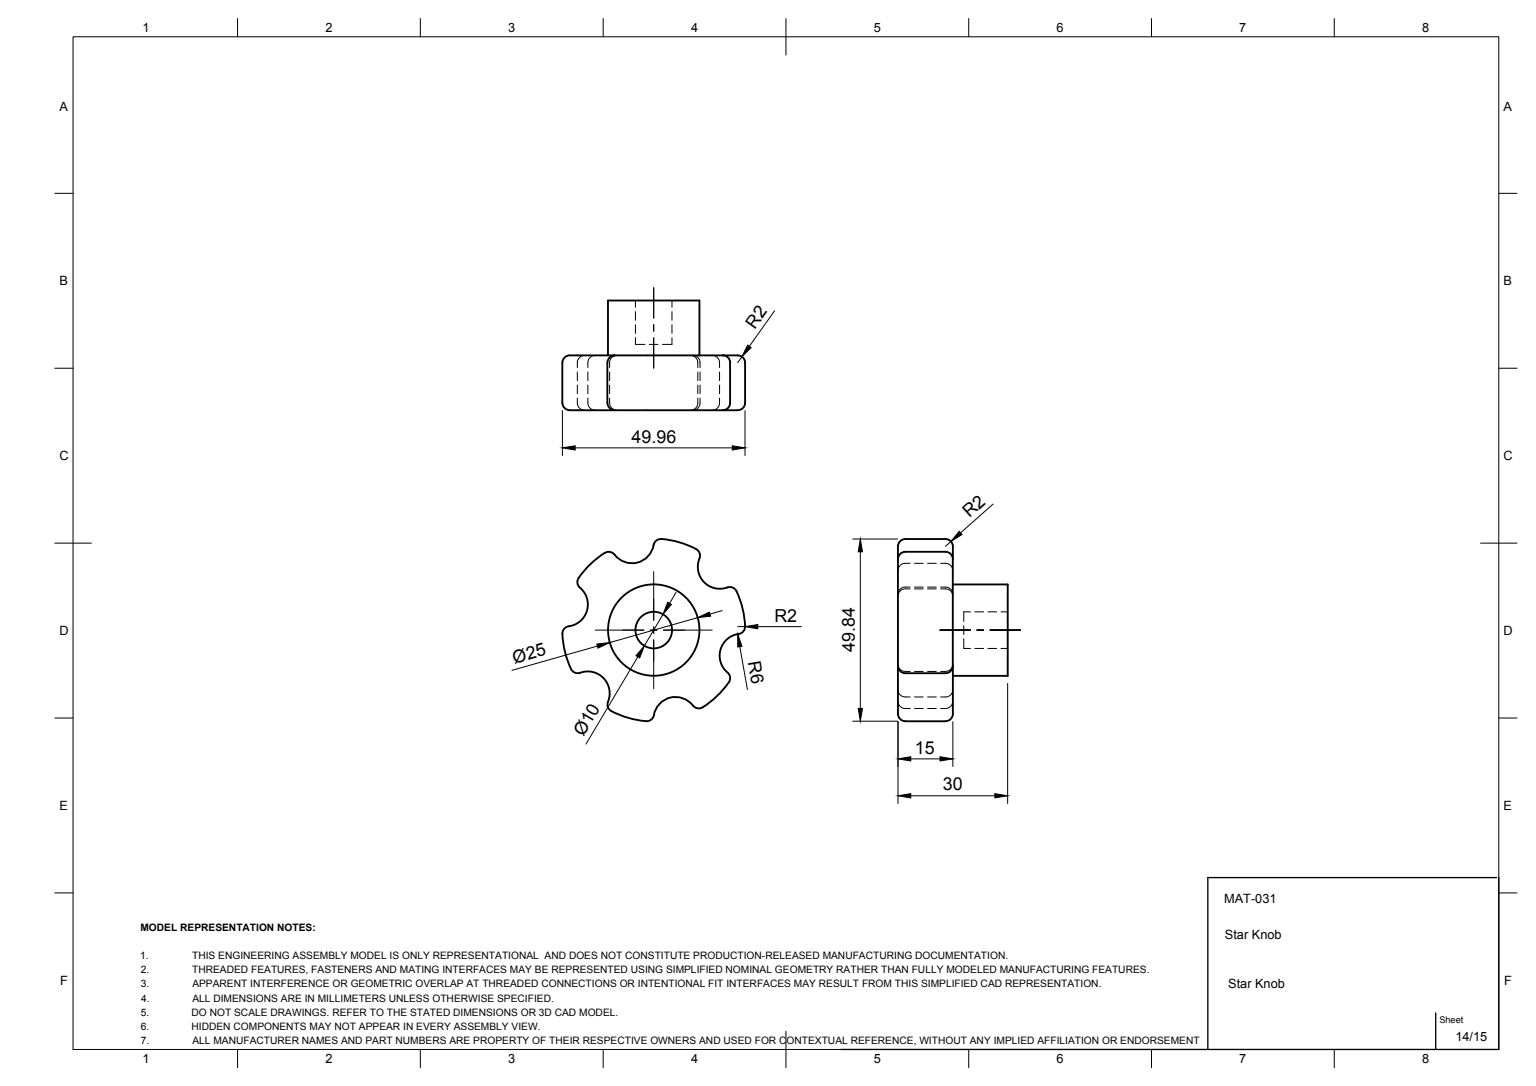
ISO-10303-21;
HEADER;
/* Generated by software containing ST-Developer
 * from STEP Tools, Inc. (www.steptools.com) 
 */

FILE_DESCRIPTION(
/* description */ ('STEP AP214'),
/* implementation_level */ '2;1');

FILE_NAME(
/* name */ 'Star Knob.step',
/* time_stamp */ '2026-11-14T06:58:01-08:00',
/* author */ (''),
/* organization */ (''),
/* preprocessor_version */ 'ST-DEVELOPER v20.2',
/* originating_system */ 'Autodesk Translation Framework v15.17.0.0',
/* authorisation */ '');

FILE_SCHEMA (('AUTOMOTIVE_DESIGN { 1 0 10303 214 3 1 1 }'));
ENDSEC;

DATA;
#10=MECHANICAL_DESIGN_GEOMETRIC_PRESENTATION_REPRESENTATION('',(#1158),#38635);
#93=SPHERICAL_SURFACE('',#18381,2.);
#94=SPHERICAL_SURFACE('',#18383,2.);
#95=SPHERICAL_SURFACE('',#18386,2.);
#96=SPHERICAL_SURFACE('',#18388,2.);
#97=SPHERICAL_SURFACE('',#18394,2.);
#98=SPHERICAL_SURFACE('',#18395,2.);
#99=SPHERICAL_SURFACE('',#18399,2.);
#100=SPHERICAL_SURFACE('',#18400,2.);
#101=SPHERICAL_SURFACE('',#18404,2.);
#102=SPHERICAL_SURFACE('',#18405,2.);
#103=SPHERICAL_SURFACE('',#18409,2.);
#104=SPHERICAL_SURFACE('',#18410,2.);
#105=SPHERICAL_SURFACE('',#18414,2.);
#106=SPHERICAL_SURFACE('',#18416,2.);
#107=SPHERICAL_SURFACE('',#18422,2.);
#108=SPHERICAL_SURFACE('',#18423,2.);
#109=SPHERICAL_SURFACE('',#18424,2.);
#110=SPHERICAL_SURFACE('',#18425,2.);
#111=SPHERICAL_SURFACE('',#18429,2.);
#112=SPHERICAL_SURFACE('',#18431,2.);
#113=SPHERICAL_SURFACE('',#18434,2.);
#114=SPHERICAL_SURFACE('',#18436,2.);
#115=SPHERICAL_SURFACE('',#18442,2.);
#116=SPHERICAL_SURFACE('',#18444,2.);
#155=TOROIDAL_SURFACE('',#18245,8.00000000000022,2.);
#156=TOROIDAL_SURFACE('',#18253,8.,2.);
#157=TOROIDAL_SURFACE('',#18258,8.00000000000095,2.);
#158=TOROIDAL_SURFACE('',#18266,8.00000000000152,2.);
#159=TOROIDAL_SURFACE('',#18274,8.00000000000143,2.);
#160=TOROIDAL_SURFACE('',#18279,8.00000000000082,2.);
#161=TOROIDAL_SURFACE('',#18314,23.,2.);
#162=TOROIDAL_SURFACE('',#18318,23.,2.);
#163=TOROIDAL_SURFACE('',#18322,23.,2.);
#164=TOROIDAL_SURFACE('',#18326,23.,2.);
#165=TOROIDAL_SURFACE('',#18330,23.,2.);
#166=TOROIDAL_SURFACE('',#18335,23.,2.);
#167=TOROIDAL_SURFACE('',#18339,23.,2.);
#168=TOROIDAL_SURFACE('',#18343,23.,2.);
#169=TOROIDAL_SURFACE('',#18347,23.,2.);
#170=TOROIDAL_SURFACE('',#18351,23.,2.);
#171=TOROIDAL_SURFACE('',#18369,23.,2.);
#172=TOROIDAL_SURFACE('',#18372,23.,2.);
#173=TOROIDAL_SURFACE('',#18384,8.00000000000082,2.);
#174=TOROIDAL_SURFACE('',#18397,8.00000000000143,2.);
#175=TOROIDAL_SURFACE('',#18407,8.00000000000152,2.);
#176=TOROIDAL_SURFACE('',#18411,8.00000000000095,2.);
#177=TOROIDAL_SURFACE('',#18433,8.,2.);
#178=TOROIDAL_SURFACE('',#18446,8.00000000000022,2.);
#883=FACE_BOUND('',#2951,.T.);
#884=FACE_BOUND('',#2953,.T.);
#1124=SHAPE_REPRESENTATION_RELATIONSHIP('SRR','None',#38697,#1138);
#1138=ADVANCED_BREP_SHAPE_REPRESENTATION('',(#1184),#38633);
#1158=STYLED_ITEM('',(#38765),#1184);
#1184=MANIFOLD_SOLID_BREP('Body1',#17624);
#1275=PLANE('',#18356);
#1276=PLANE('',#18362);
#1277=PLANE('',#18367);
#1278=PLANE('',#18368);
#1891=FACE_OUTER_BOUND('',#2918,.T.);
#1892=FACE_OUTER_BOUND('',#2919,.T.);
#1893=FACE_OUTER_BOUND('',#2920,.T.);
#1894=FACE_OUTER_BOUND('',#2921,.T.);
#1895=FACE_OUTER_BOUND('',#2922,.T.);
#1896=FACE_OUTER_BOUND('',#2923,.T.);
#1897=FACE_OUTER_BOUND('',#2924,.T.);
#1898=FACE_OUTER_BOUND('',#2925,.T.);
#1899=FACE_OUTER_BOUND('',#2926,.T.);
#1900=FACE_OUTER_BOUND('',#2927,.T.);
#1901=FACE_OUTER_BOUND('',#2928,.T.);
#1902=FACE_OUTER_BOUND('',#2929,.T.);
#1903=FACE_OUTER_BOUND('',#2930,.T.);
#1904=FACE_OUTER_BOUND('',#2931,.T.);
#1905=FACE_OUTER_BOUND('',#2932,.T.);
#1906=FACE_OUTER_BOUND('',#2933,.T.);
#1907=FACE_OUTER_BOUND('',#2934,.T.);
#1908=FACE_OUTER_BOUND('',#2935,.T.);
#1909=FACE_OUTER_BOUND('',#2936,.T.);
#1910=FACE_OUTER_BOUND('',#2937,.T.);
#1911=FACE_OUTER_BOUND('',#2938,.T.);
#1912=FACE_OUTER_BOUND('',#2939,.T.);
#1913=FACE_OUTER_BOUND('',#2940,.T.);
#1914=FACE_OUTER_BOUND('',#2941,.T.);
#1915=FACE_OUTER_BOUND('',#2942,.T.);
#1916=FACE_OUTER_BOUND('',#2943,.T.);
#1917=FACE_OUTER_BOUND('',#2944,.T.);
#1918=FACE_OUTER_BOUND('',#2945,.T.);
#1919=FACE_OUTER_BOUND('',#2946,.T.);
#1920=FACE_OUTER_BOUND('',#2947,.T.);
#1921=FACE_OUTER_BOUND('',#2948,.T.);
#1922=FACE_OUTER_BOUND('',#2949,.T.);
#1923=FACE_OUTER_BOUND('',#2950,.T.);
#1924=FACE_OUTER_BOUND('',#2952,.T.);
#1925=FACE_OUTER_BOUND('',#2954,.T.);
#1926=FACE_OUTER_BOUND('',#2955,.T.);
#1927=FACE_OUTER_BOUND('',#2956,.T.);
#1928=FACE_OUTER_BOUND('',#2957,.T.);
#1929=FACE_OUTER_BOUND('',#2958,.T.);
#1930=FACE_OUTER_BOUND('',#2959,.T.);
#1931=FACE_OUTER_BOUND('',#2960,.T.);
#1932=FACE_OUTER_BOUND('',#2961,.T.);
#1933=FACE_OUTER_BOUND('',#2962,.T.);
#1934=FACE_OUTER_BOUND('',#2963,.T.);
#1935=FACE_OUTER_BOUND('',#2964,.T.);
#1936=FACE_OUTER_BOUND('',#2965,.T.);
#1937=FACE_OUTER_BOUND('',#2966,.T.);
#1938=FACE_OUTER_BOUND('',#2967,.T.);
#1939=FACE_OUTER_BOUND('',#2968,.T.);
#1940=FACE_OUTER_BOUND('',#2969,.T.);
#1941=FACE_OUTER_BOUND('',#2970,.T.);
#1942=FACE_OUTER_BOUND('',#2971,.T.);
#1943=FACE_OUTER_BOUND('',#2972,.T.);
#1944=FACE_OUTER_BOUND('',#2973,.T.);
#1945=FACE_OUTER_BOUND('',#2974,.T.);
#1946=FACE_OUTER_BOUND('',#2975,.T.);
#1947=FACE_OUTER_BOUND('',#2976,.T.);
#1948=FACE_OUTER_BOUND('',#2977,.T.);
#1949=FACE_OUTER_BOUND('',#2978,.T.);
#1950=FACE_OUTER_BOUND('',#2979,.T.);
#1951=FACE_OUTER_BOUND('',#2980,.T.);
#1952=FACE_OUTER_BOUND('',#2981,.T.);
#1953=FACE_OUTER_BOUND('',#2982,.T.);
#1954=FACE_OUTER_BOUND('',#2983,.T.);
#1955=FACE_OUTER_BOUND('',#2984,.T.);
#1956=FACE_OUTER_BOUND('',#2985,.T.);
#1957=FACE_OUTER_BOUND('',#2986,.T.);
#1958=FACE_OUTER_BOUND('',#2987,.T.);
#1959=FACE_OUTER_BOUND('',#2988,.T.);
#1960=FACE_OUTER_BOUND('',#2989,.T.);
#1961=FACE_OUTER_BOUND('',#2990,.T.);
#1962=FACE_OUTER_BOUND('',#2991,.T.);
#1963=FACE_OUTER_BOUND('',#2992,.T.);
#1964=FACE_OUTER_BOUND('',#2993,.T.);
#1965=FACE_OUTER_BOUND('',#2994,.T.);
#1966=FACE_OUTER_BOUND('',#2995,.T.);
#1967=FACE_OUTER_BOUND('',#2996,.T.);
#1968=FACE_OUTER_BOUND('',#2997,.T.);
#2918=EDGE_LOOP('',(#12069,#12070,#12071,#12072));
#2919=EDGE_LOOP('',(#12073,#12074,#12075,#12076));
#2920=EDGE_LOOP('',(#12077,#12078,#12079,#12080));
#2921=EDGE_LOOP('',(#12081,#12082,#12083,#12084));
#2922=EDGE_LOOP('',(#12085,#12086,#12087,#12088));
#2923=EDGE_LOOP('',(#12089,#12090,#12091,#12092));
#2924=EDGE_LOOP('',(#12093,#12094,#12095,#12096));
#2925=EDGE_LOOP('',(#12097,#12098,#12099,#12100));
#2926=EDGE_LOOP('',(#12101,#12102,#12103,#12104));
#2927=EDGE_LOOP('',(#12105,#12106,#12107,#12108));
#2928=EDGE_LOOP('',(#12109,#12110,#12111,#12112));
#2929=EDGE_LOOP('',(#12113,#12114,#12115,#12116));
#2930=EDGE_LOOP('',(#12117,#12118,#12119,#12120));
#2931=EDGE_LOOP('',(#12121,#12122,#12123,#12124));
#2932=EDGE_LOOP('',(#12125,#12126,#12127,#12128));
#2933=EDGE_LOOP('',(#12129,#12130,#12131,#12132));
#2934=EDGE_LOOP('',(#12133,#12134,#12135,#12136));
#2935=EDGE_LOOP('',(#12137,#12138,#12139,#12140));
#2936=EDGE_LOOP('',(#12141,#12142,#12143,#12144));
#2937=EDGE_LOOP('',(#12145,#12146,#12147,#12148));
#2938=EDGE_LOOP('',(#12149,#12150,#12151,#12152));
#2939=EDGE_LOOP('',(#12153,#12154,#12155,#12156));
#2940=EDGE_LOOP('',(#12157,#12158,#12159,#12160));
#2941=EDGE_LOOP('',(#12161,#12162,#12163,#12164));
#2942=EDGE_LOOP('',(#12165,#12166,#12167,#12168));
#2943=EDGE_LOOP('',(#12169,#12170,#12171,#12172));
#2944=EDGE_LOOP('',(#12173,#12174,#12175,#12176));
#2945=EDGE_LOOP('',(#12177,#12178,#12179,#12180));
#2946=EDGE_LOOP('',(#12181,#12182,#12183,#12184));
#2947=EDGE_LOOP('',(#12185,#12186,#12187,#12188));
#2948=EDGE_LOOP('',(#12189,#12190,#12191,#12192,#12193,#12194,#12195,#12196,
#12197,#12198,#12199,#12200));
#2949=EDGE_LOOP('',(#12201,#12202,#12203,#12204));
#2950=EDGE_LOOP('',(#12205,#12206,#12207,#12208,#12209,#12210,#12211,#12212,
#12213,#12214,#12215,#12216));
#2951=EDGE_LOOP('',(#12217));
#2952=EDGE_LOOP('',(#12218));
#2953=EDGE_LOOP('',(#12219));
#2954=EDGE_LOOP('',(#12220));
#2955=EDGE_LOOP('',(#12221,#12222,#12223,#12224));
#2956=EDGE_LOOP('',(#12225,#12226,#12227,#12228));
#2957=EDGE_LOOP('',(#12229,#12230,#12231,#12232));
#2958=EDGE_LOOP('',(#12233,#12234,#12235,#12236));
#2959=EDGE_LOOP('',(#12237,#12238,#12239,#12240));
#2960=EDGE_LOOP('',(#12241,#12242,#12243));
#2961=EDGE_LOOP('',(#12244,#12245,#12246));
#2962=EDGE_LOOP('',(#12247,#12248,#12249,#12250));
#2963=EDGE_LOOP('',(#12251,#12252,#12253));
#2964=EDGE_LOOP('',(#12254,#12255,#12256));
#2965=EDGE_LOOP('',(#12257,#12258,#12259,#12260));
#2966=EDGE_LOOP('',(#12261,#12262,#12263,#12264));
#2967=EDGE_LOOP('',(#12265,#12266,#12267));
#2968=EDGE_LOOP('',(#12268,#12269,#12270));
#2969=EDGE_LOOP('',(#12271,#12272,#12273,#12274));
#2970=EDGE_LOOP('',(#12275,#12276,#12277));
#2971=EDGE_LOOP('',(#12278,#12279,#12280));
#2972=EDGE_LOOP('',(#12281,#12282,#12283,#12284));
#2973=EDGE_LOOP('',(#12285,#12286,#12287));
#2974=EDGE_LOOP('',(#12288,#12289,#12290));
#2975=EDGE_LOOP('',(#12291,#12292,#12293,#12294));
#2976=EDGE_LOOP('',(#12295,#12296,#12297));
#2977=EDGE_LOOP('',(#12298,#12299,#12300));
#2978=EDGE_LOOP('',(#12301,#12302,#12303,#12304));
#2979=EDGE_LOOP('',(#12305,#12306,#12307));
#2980=EDGE_LOOP('',(#12308,#12309,#12310));
#2981=EDGE_LOOP('',(#12311,#12312,#12313,#12314));
#2982=EDGE_LOOP('',(#12315,#12316,#12317,#12318));
#2983=EDGE_LOOP('',(#12319,#12320,#12321));
#2984=EDGE_LOOP('',(#12322,#12323,#12324));
#2985=EDGE_LOOP('',(#12325,#12326,#12327));
#2986=EDGE_LOOP('',(#12328,#12329,#12330));
#2987=EDGE_LOOP('',(#12331,#12332,#12333,#12334));
#2988=EDGE_LOOP('',(#12335,#12336,#12337));
#2989=EDGE_LOOP('',(#12338,#12339,#12340));
#2990=EDGE_LOOP('',(#12341,#12342,#12343,#12344));
#2991=EDGE_LOOP('',(#12345,#12346,#12347));
#2992=EDGE_LOOP('',(#12348,#12349,#12350));
#2993=EDGE_LOOP('',(#12351,#12352,#12353,#12354));
#2994=EDGE_LOOP('',(#12355,#12356,#12357,#12358));
#2995=EDGE_LOOP('',(#12359,#12360,#12361));
#2996=EDGE_LOOP('',(#12362,#12363,#12364));
#2997=EDGE_LOOP('',(#12365,#12366,#12367,#12368));
#3918=LINE('',#33069,#4862);
#3919=LINE('',#33072,#4863);
#3920=LINE('',#33095,#4864);
#3921=LINE('',#33098,#4865);
#3922=LINE('',#33112,#4866);
#3923=LINE('',#33115,#4867);
#3924=LINE('',#33138,#4868);
#3925=LINE('',#33140,#4869);
#3926=LINE('',#33143,#4870);
#3927=LINE('',#33147,#4871);
#3928=LINE('',#33151,#4872);
#3929=LINE('',#33154,#4873);
#3930=LINE('',#33159,#4874);
#3931=LINE('',#33165,#4875);
#3932=LINE('',#33172,#4876);
#3933=LINE('',#33175,#4877);
#3934=LINE('',#33180,#4878);
#3935=LINE('',#33189,#4879);
#3936=LINE('',#33196,#4880);
#3937=LINE('',#33199,#4881);
#3938=LINE('',#33262,#4882);
#3939=LINE('',#33263,#4883);
#3940=LINE('',#33281,#4884);
#3941=LINE('',#33284,#4885);
#3942=LINE('',#33287,#4886);
#3943=LINE('',#33291,#4887);
#4862=VECTOR('',#20893,1000.);
#4863=VECTOR('',#20896,1000.);
#4864=VECTOR('',#20921,1000.);
#4865=VECTOR('',#20924,1000.);
#4866=VECTOR('',#20939,1000.);
#4867=VECTOR('',#20942,1000.);
#4868=VECTOR('',#20967,1000.);
#4869=VECTOR('',#20970,1000.);
#4870=VECTOR('',#20973,1000.);
#4871=VECTOR('',#20978,1000.);
#4872=VECTOR('',#20983,1000.);
#4873=VECTOR('',#20986,1000.);
#4874=VECTOR('',#20991,5.);
#4875=VECTOR('',#20998,12.5);
#4876=VECTOR('',#21005,1000.);
#4877=VECTOR('',#21008,1000.);
#4878=VECTOR('',#21013,1000.);
#4879=VECTOR('',#21026,1000.);
#4880=VECTOR('',#21033,1000.);
#4881=VECTOR('',#21036,1000.);
#4882=VECTOR('',#21133,1000.);
#4883=VECTOR('',#21134,1000.);
#4884=VECTOR('',#21163,1000.);
#4885=VECTOR('',#21166,1000.);
#4886=VECTOR('',#21169,1000.);
#4887=VECTOR('',#21174,1000.);
#5795=CIRCLE('',#18246,6.00000000000022);
#5796=CIRCLE('',#18247,2.);
#5797=CIRCLE('',#18248,8.00000000000022);
#5798=CIRCLE('',#18249,2.);
#5799=CIRCLE('',#18251,2.);
#5800=CIRCLE('',#18252,2.);
#5801=CIRCLE('',#18254,6.);
#5802=CIRCLE('',#18255,2.);
#5803=CIRCLE('',#18256,8.);
#5804=CIRCLE('',#18257,2.);
#5805=CIRCLE('',#18259,6.00000000000095);
#5806=CIRCLE('',#18260,2.);
#5807=CIRCLE('',#18261,8.00000000000095);
#5808=CIRCLE('',#18262,2.);
#5809=CIRCLE('',#18264,2.);
#5810=CIRCLE('',#18265,2.);
#5811=CIRCLE('',#18267,6.00000000000152);
#5812=CIRCLE('',#18268,2.);
#5813=CIRCLE('',#18269,8.00000000000152);
#5814=CIRCLE('',#18270,2.);
#5815=CIRCLE('',#18272,2.);
#5816=CIRCLE('',#18273,2.);
#5817=CIRCLE('',#18275,6.00000000000143);
#5818=CIRCLE('',#18276,2.);
#5819=CIRCLE('',#18277,8.00000000000143);
#5820=CIRCLE('',#18278,2.);
#5821=CIRCLE('',#18280,6.00000000000081);
#5822=CIRCLE('',#18281,2.);
#5823=CIRCLE('',#18282,8.00000000000082);
#5824=CIRCLE('',#18283,2.);
#5825=CIRCLE('',#18285,2.);
#5826=CIRCLE('',#18286,2.);
#5827=CIRCLE('',#18288,6.00000000000143);
#5828=CIRCLE('',#18290,6.00000000000152);
#5829=CIRCLE('',#18292,6.00000000000095);
#5830=CIRCLE('',#18294,5.);
#5831=CIRCLE('',#18295,5.);
#5832=CIRCLE('',#18297,12.5);
#5833=CIRCLE('',#18298,12.5);
#5834=CIRCLE('',#18300,25.);
#5835=CIRCLE('',#18301,25.);
#5836=CIRCLE('',#18303,25.);
#5837=CIRCLE('',#18304,25.);
#5838=CIRCLE('',#18306,25.);
#5839=CIRCLE('',#18307,25.);
#5840=CIRCLE('',#18309,25.);
#5841=CIRCLE('',#18310,25.);
#5842=CIRCLE('',#18312,25.);
#5843=CIRCLE('',#18313,25.);
#5844=CIRCLE('',#18315,23.);
#5845=CIRCLE('',#18316,2.);
#5846=CIRCLE('',#18317,2.);
#5847=CIRCLE('',#18319,23.);
#5848=CIRCLE('',#18320,2.);
#5849=CIRCLE('',#18321,2.);
#5850=CIRCLE('',#18323,2.);
#5851=CIRCLE('',#18324,23.);
#5852=CIRCLE('',#18325,2.);
#5853=CIRCLE('',#18327,2.);
#5854=CIRCLE('',#18328,23.);
#5855=CIRCLE('',#18329,2.);
#5856=CIRCLE('',#18331,25.);
#5857=CIRCLE('',#18332,2.);
#5858=CIRCLE('',#18333,23.);
#5859=CIRCLE('',#18334,2.);
#5860=CIRCLE('',#18336,2.);
#5861=CIRCLE('',#18337,23.);
#5862=CIRCLE('',#18338,2.);
#5863=CIRCLE('',#18340,2.);
#5864=CIRCLE('',#18341,23.);
#5865=CIRCLE('',#18342,2.);
#5866=CIRCLE('',#18344,23.);
#5867=CIRCLE('',#18345,2.);
#5868=CIRCLE('',#18346,2.);
#5869=CIRCLE('',#18348,23.);
#5870=CIRCLE('',#18349,2.);
#5871=CIRCLE('',#18350,2.);
#5872=CIRCLE('',#18352,23.);
#5873=CIRCLE('',#18353,2.);
#5874=CIRCLE('',#18354,25.);
#5875=CIRCLE('',#18355,2.);
#5876=CIRCLE('',#18357,8.00000000000082);
#5877=CIRCLE('',#18358,8.);
#5878=CIRCLE('',#18359,8.00000000000022);
#5879=CIRCLE('',#18360,23.);
#5880=CIRCLE('',#18363,8.00000000000143);
#5881=CIRCLE('',#18364,8.00000000000151);
#5882=CIRCLE('',#18365,23.);
#5883=CIRCLE('',#18366,8.00000000000095);
#5884=CIRCLE('',#18370,2.);
#5885=CIRCLE('',#18371,2.);
#5886=CIRCLE('',#18373,2.);
#5887=CIRCLE('',#18374,2.);
#5888=CIRCLE('',#18376,6.00000000000022);
#5889=CIRCLE('',#18378,6.00000000000081);
#5890=CIRCLE('',#18380,6.);
#5891=CIRCLE('',#18382,2.);
#5892=CIRCLE('',#18385,2.);
#5893=CIRCLE('',#18387,2.);
#5894=CIRCLE('',#18389,2.);
#5895=CIRCLE('',#18392,2.);
#5896=CIRCLE('',#18393,2.);
#5897=CIRCLE('',#18396,2.);
#5898=CIRCLE('',#18398,2.);
#5899=CIRCLE('',#18402,2.);
#5900=CIRCLE('',#18403,2.);
#5901=CIRCLE('',#18406,2.);
#5902=CIRCLE('',#18408,2.);
#5903=CIRCLE('',#18412,2.);
#5904=CIRCLE('',#18413,2.);
#5905=CIRCLE('',#18415,2.);
#5906=CIRCLE('',#18417,2.);
#5907=CIRCLE('',#18419,2.);
#5908=CIRCLE('',#18421,2.);
#5909=CIRCLE('',#18426,2.);
#5910=CIRCLE('',#18428,2.);
#5911=CIRCLE('',#18430,2.);
#5912=CIRCLE('',#18432,2.);
#5913=CIRCLE('',#18435,2.);
#5914=CIRCLE('',#18437,2.);
#5915=CIRCLE('',#18439,2.);
#5916=CIRCLE('',#18441,2.);
#5917=CIRCLE('',#18443,2.);
#5918=CIRCLE('',#18445,2.);
#6885=VERTEX_POINT('',#33056);
#6886=VERTEX_POINT('',#33057);
#6887=VERTEX_POINT('',#33059);
#6888=VERTEX_POINT('',#33061);
#6889=VERTEX_POINT('',#33065);
#6890=VERTEX_POINT('',#33066);
#6891=VERTEX_POINT('',#33068);
#6892=VERTEX_POINT('',#33070);
#6893=VERTEX_POINT('',#33074);
#6894=VERTEX_POINT('',#33076);
#6895=VERTEX_POINT('',#33078);
#6896=VERTEX_POINT('',#33082);
#6897=VERTEX_POINT('',#33083);
#6898=VERTEX_POINT('',#33085);
#6899=VERTEX_POINT('',#33087);
#6900=VERTEX_POINT('',#33091);
#6901=VERTEX_POINT('',#33092);
#6902=VERTEX_POINT('',#33094);
#6903=VERTEX_POINT('',#33096);
#6904=VERTEX_POINT('',#33100);
#6905=VERTEX_POINT('',#33102);
#6906=VERTEX_POINT('',#33104);
#6907=VERTEX_POINT('',#33108);
#6908=VERTEX_POINT('',#33109);
#6909=VERTEX_POINT('',#33111);
#6910=VERTEX_POINT('',#33113);
#6911=VERTEX_POINT('',#33117);
#6912=VERTEX_POINT('',#33119);
#6913=VERTEX_POINT('',#33121);
#6914=VERTEX_POINT('',#33125);
#6915=VERTEX_POINT('',#33126);
#6916=VERTEX_POINT('',#33128);
#6917=VERTEX_POINT('',#33130);
#6918=VERTEX_POINT('',#33134);
#6919=VERTEX_POINT('',#33135);
#6920=VERTEX_POINT('',#33137);
#6921=VERTEX_POINT('',#33142);
#6922=VERTEX_POINT('',#33146);
#6923=VERTEX_POINT('',#33150);
#6924=VERTEX_POINT('',#33152);
#6925=VERTEX_POINT('',#33156);
#6926=VERTEX_POINT('',#33158);
#6927=VERTEX_POINT('',#33162);
#6928=VERTEX_POINT('',#33164);
#6929=VERTEX_POINT('',#33168);
#6930=VERTEX_POINT('',#33169);
#6931=VERTEX_POINT('',#33171);
#6932=VERTEX_POINT('',#33173);
#6933=VERTEX_POINT('',#33177);
#6934=VERTEX_POINT('',#33179);
#6935=VERTEX_POINT('',#33186);
#6936=VERTEX_POINT('',#33188);
#6937=VERTEX_POINT('',#33192);
#6938=VERTEX_POINT('',#33193);
#6939=VERTEX_POINT('',#33195);
#6940=VERTEX_POINT('',#33197);
#6941=VERTEX_POINT('',#33201);
#6942=VERTEX_POINT('',#33202);
#6943=VERTEX_POINT('',#33207);
#6944=VERTEX_POINT('',#33208);
#6945=VERTEX_POINT('',#33213);
#6946=VERTEX_POINT('',#33222);
#6947=VERTEX_POINT('',#33223);
#6948=VERTEX_POINT('',#33226);
#6949=VERTEX_POINT('',#33238);
#6950=VERTEX_POINT('',#33243);
#6951=VERTEX_POINT('',#33244);
#6952=VERTEX_POINT('',#33249);
#6953=VERTEX_POINT('',#33251);
#6954=VERTEX_POINT('',#33253);
#6955=VERTEX_POINT('',#33266);
#6956=VERTEX_POINT('',#33268);
#6957=VERTEX_POINT('',#33280);
#6958=VERTEX_POINT('',#33282);
#6959=VERTEX_POINT('',#33286);
#6960=VERTEX_POINT('',#33290);
#8821=EDGE_CURVE('',#6885,#6886,#5795,.T.);
#8822=EDGE_CURVE('',#6887,#6885,#5796,.T.);
#8823=EDGE_CURVE('',#6888,#6887,#5797,.T.);
#8824=EDGE_CURVE('',#6886,#6888,#5798,.T.);
#8825=EDGE_CURVE('',#6889,#6890,#5799,.T.);
#8826=EDGE_CURVE('',#6891,#6889,#3918,.T.);
#8827=EDGE_CURVE('',#6891,#6892,#5800,.T.);
#8828=EDGE_CURVE('',#6890,#6892,#3919,.T.);
#8829=EDGE_CURVE('',#6892,#6893,#5801,.T.);
#8830=EDGE_CURVE('',#6894,#6892,#5802,.T.);
#8831=EDGE_CURVE('',#6895,#6894,#5803,.T.);
#8832=EDGE_CURVE('',#6893,#6895,#5804,.T.);
#8833=EDGE_CURVE('',#6896,#6897,#5805,.T.);
#8834=EDGE_CURVE('',#6896,#6898,#5806,.T.);
#8835=EDGE_CURVE('',#6899,#6898,#5807,.T.);
#8836=EDGE_CURVE('',#6899,#6897,#5808,.T.);
#8837=EDGE_CURVE('',#6900,#6901,#5809,.T.);
#8838=EDGE_CURVE('',#6902,#6901,#3920,.T.);
#8839=EDGE_CURVE('',#6902,#6903,#5810,.T.);
#8840=EDGE_CURVE('',#6900,#6903,#3921,.T.);
#8841=EDGE_CURVE('',#6903,#6904,#5811,.T.);
#8842=EDGE_CURVE('',#6905,#6903,#5812,.T.);
#8843=EDGE_CURVE('',#6906,#6905,#5813,.T.);
#8844=EDGE_CURVE('',#6906,#6904,#5814,.T.);
#8845=EDGE_CURVE('',#6907,#6908,#5815,.T.);
#8846=EDGE_CURVE('',#6909,#6908,#3922,.T.);
#8847=EDGE_CURVE('',#6909,#6910,#5816,.T.);
#8848=EDGE_CURVE('',#6907,#6910,#3923,.T.);
#8849=EDGE_CURVE('',#6910,#6911,#5817,.T.);
#8850=EDGE_CURVE('',#6912,#6910,#5818,.T.);
#8851=EDGE_CURVE('',#6913,#6912,#5819,.T.);
#8852=EDGE_CURVE('',#6913,#6911,#5820,.T.);
#8853=EDGE_CURVE('',#6914,#6915,#5821,.T.);
#8854=EDGE_CURVE('',#6914,#6916,#5822,.T.);
#8855=EDGE_CURVE('',#6917,#6916,#5823,.T.);
#8856=EDGE_CURVE('',#6915,#6917,#5824,.T.);
#8857=EDGE_CURVE('',#6918,#6919,#5825,.T.);
#8858=EDGE_CURVE('',#6920,#6918,#3924,.T.);
#8859=EDGE_CURVE('',#6914,#6920,#5826,.T.);
#8860=EDGE_CURVE('',#6919,#6914,#3925,.T.);
#8861=EDGE_CURVE('',#6911,#6921,#3926,.T.);
#8862=EDGE_CURVE('',#6921,#6907,#5827,.T.);
#8863=EDGE_CURVE('',#6904,#6922,#3927,.T.);
#8864=EDGE_CURVE('',#6922,#6900,#5828,.T.);
#8865=EDGE_CURVE('',#6897,#6923,#3928,.T.);
#8866=EDGE_CURVE('',#6923,#6924,#5829,.T.);
#8867=EDGE_CURVE('',#6924,#6896,#3929,.T.);
#8868=EDGE_CURVE('',#6925,#6925,#5830,.T.);
#8869=EDGE_CURVE('',#6925,#6926,#3930,.T.);
#8870=EDGE_CURVE('',#6926,#6926,#5831,.T.);
#8871=EDGE_CURVE('',#6927,#6927,#5832,.T.);
#8872=EDGE_CURVE('',#6927,#6928,#3931,.T.);
#8873=EDGE_CURVE('',#6928,#6928,#5833,.T.);
#8874=EDGE_CURVE('',#6929,#6930,#5834,.T.);
#8875=EDGE_CURVE('',#6930,#6931,#3932,.T.);
#8876=EDGE_CURVE('',#6931,#6932,#5835,.T.);
#8877=EDGE_CURVE('',#6932,#6929,#3933,.T.);
#8878=EDGE_CURVE('',#6889,#6933,#5836,.T.);
#8879=EDGE_CURVE('',#6933,#6934,#3934,.T.);
#8880=EDGE_CURVE('',#6934,#6891,#5837,.T.);
#8881=EDGE_CURVE('',#6908,#6920,#5838,.T.);
#8882=EDGE_CURVE('',#6918,#6909,#5839,.T.);
#8883=EDGE_CURVE('',#6901,#6935,#5840,.T.);
#8884=EDGE_CURVE('',#6935,#6936,#3935,.T.);
#8885=EDGE_CURVE('',#6936,#6902,#5841,.T.);
#8886=EDGE_CURVE('',#6937,#6938,#5842,.T.);
#8887=EDGE_CURVE('',#6938,#6939,#3936,.T.);
#8888=EDGE_CURVE('',#6939,#6940,#5843,.T.);
#8889=EDGE_CURVE('',#6940,#6937,#3937,.T.);
#8890=EDGE_CURVE('',#6941,#6942,#5844,.T.);
#8891=EDGE_CURVE('',#6941,#6933,#5845,.T.);
#8892=EDGE_CURVE('',#6889,#6942,#5846,.T.);
#8893=EDGE_CURVE('',#6943,#6944,#5847,.T.);
#8894=EDGE_CURVE('',#6943,#6930,#5848,.T.);
#8895=EDGE_CURVE('',#6929,#6944,#5849,.T.);
#8896=EDGE_CURVE('',#6918,#6945,#5850,.T.);
#8897=EDGE_CURVE('',#6912,#6945,#5851,.T.);
#8898=EDGE_CURVE('',#6912,#6909,#5852,.T.);
#8899=EDGE_CURVE('',#6936,#6913,#5853,.T.);
#8900=EDGE_CURVE('',#6905,#6913,#5854,.T.);
#8901=EDGE_CURVE('',#6905,#6902,#5855,.T.);
#8902=EDGE_CURVE('',#6946,#6947,#5856,.T.);
#8903=EDGE_CURVE('',#6946,#6899,#5857,.T.);
#8904=EDGE_CURVE('',#6948,#6899,#5858,.T.);
#8905=EDGE_CURVE('',#6948,#6947,#5859,.T.);
#8906=EDGE_CURVE('',#6934,#6917,#5860,.T.);
#8907=EDGE_CURVE('',#6894,#6917,#5861,.T.);
#8908=EDGE_CURVE('',#6894,#6891,#5862,.T.);
#8909=EDGE_CURVE('',#6931,#6895,#5863,.T.);
#8910=EDGE_CURVE('',#6887,#6895,#5864,.T.);
#8911=EDGE_CURVE('',#6887,#6932,#5865,.T.);
#8912=EDGE_CURVE('',#6916,#6949,#5866,.T.);
#8913=EDGE_CURVE('',#6916,#6920,#5867,.T.);
#8914=EDGE_CURVE('',#6908,#6949,#5868,.T.);
#8915=EDGE_CURVE('',#6950,#6951,#5869,.T.);
#8916=EDGE_CURVE('',#6950,#6935,#5870,.T.);
#8917=EDGE_CURVE('',#6901,#6951,#5871,.T.);
#8918=EDGE_CURVE('',#6952,#6888,#5872,.T.);
#8919=EDGE_CURVE('',#6952,#6953,#5873,.T.);
#8920=EDGE_CURVE('',#6954,#6953,#5874,.T.);
#8921=EDGE_CURVE('',#6954,#6888,#5875,.T.);
#8922=EDGE_CURVE('',#6945,#6941,#5876,.T.);
#8923=EDGE_CURVE('',#6942,#6943,#5877,.T.);
#8924=EDGE_CURVE('',#6944,#6948,#5878,.T.);
#8925=EDGE_CURVE('',#6898,#6906,#5879,.T.);
#8926=EDGE_CURVE('',#6953,#6946,#3938,.T.);
#8927=EDGE_CURVE('',#6947,#6954,#3939,.T.);
#8928=EDGE_CURVE('',#6949,#6950,#5880,.T.);
#8929=EDGE_CURVE('',#6951,#6955,#5881,.T.);
#8930=EDGE_CURVE('',#6955,#6956,#5882,.T.);
#8931=EDGE_CURVE('',#6956,#6952,#5883,.T.);
#8932=EDGE_CURVE('',#6939,#6906,#5884,.T.);
#8933=EDGE_CURVE('',#6898,#6940,#5885,.T.);
#8934=EDGE_CURVE('',#6955,#6938,#5886,.T.);
#8935=EDGE_CURVE('',#6937,#6956,#5887,.T.);
#8936=EDGE_CURVE('',#6886,#6957,#3940,.T.);
#8937=EDGE_CURVE('',#6957,#6958,#5888,.T.);
#8938=EDGE_CURVE('',#6958,#6885,#3941,.T.);
#8939=EDGE_CURVE('',#6915,#6959,#3942,.T.);
#8940=EDGE_CURVE('',#6959,#6919,#5889,.T.);
#8941=EDGE_CURVE('',#6893,#6960,#3943,.T.);
#8942=EDGE_CURVE('',#6960,#6890,#5890,.T.);
#8943=EDGE_CURVE('',#6945,#6919,#5891,.T.);
#8944=EDGE_CURVE('',#6941,#6959,#5892,.T.);
#8945=EDGE_CURVE('',#6933,#6959,#5893,.T.);
#8946=EDGE_CURVE('',#6915,#6934,#5894,.T.);
#8947=EDGE_CURVE('',#6936,#6911,#5895,.T.);
#8948=EDGE_CURVE('',#6921,#6935,#5896,.T.);
#8949=EDGE_CURVE('',#6921,#6950,#5897,.T.);
#8950=EDGE_CURVE('',#6907,#6949,#5898,.T.);
#8951=EDGE_CURVE('',#6939,#6904,#5899,.T.);
#8952=EDGE_CURVE('',#6922,#6938,#5900,.T.);
#8953=EDGE_CURVE('',#6922,#6955,#5901,.T.);
#8954=EDGE_CURVE('',#6900,#6951,#5902,.T.);
#8955=EDGE_CURVE('',#6952,#6923,#5903,.T.);
#8956=EDGE_CURVE('',#6924,#6956,#5904,.T.);
#8957=EDGE_CURVE('',#6953,#6923,#5905,.T.);
#8958=EDGE_CURVE('',#6924,#6937,#5906,.T.);
#8959=EDGE_CURVE('',#6946,#6897,#5907,.T.);
#8960=EDGE_CURVE('',#6896,#6940,#5908,.T.);
#8961=EDGE_CURVE('',#6893,#6931,#5909,.T.);
#8962=EDGE_CURVE('',#6960,#6930,#5910,.T.);
#8963=EDGE_CURVE('',#6942,#6890,#5911,.T.);
#8964=EDGE_CURVE('',#6960,#6943,#5912,.T.);
#8965=EDGE_CURVE('',#6932,#6885,#5913,.T.);
#8966=EDGE_CURVE('',#6886,#6954,#5914,.T.);
#8967=EDGE_CURVE('',#6929,#6958,#5915,.T.);
#8968=EDGE_CURVE('',#6957,#6947,#5916,.T.);
#8969=EDGE_CURVE('',#6944,#6958,#5917,.T.);
#8970=EDGE_CURVE('',#6957,#6948,#5918,.T.);
#12069=ORIENTED_EDGE('',*,*,#8821,.F.);
#12070=ORIENTED_EDGE('',*,*,#8822,.F.);
#12071=ORIENTED_EDGE('',*,*,#8823,.F.);
#12072=ORIENTED_EDGE('',*,*,#8824,.F.);
#12073=ORIENTED_EDGE('',*,*,#8825,.F.);
#12074=ORIENTED_EDGE('',*,*,#8826,.F.);
#12075=ORIENTED_EDGE('',*,*,#8827,.T.);
#12076=ORIENTED_EDGE('',*,*,#8828,.F.);
#12077=ORIENTED_EDGE('',*,*,#8829,.F.);
#12078=ORIENTED_EDGE('',*,*,#8830,.F.);
#12079=ORIENTED_EDGE('',*,*,#8831,.F.);
#12080=ORIENTED_EDGE('',*,*,#8832,.F.);
#12081=ORIENTED_EDGE('',*,*,#8833,.F.);
#12082=ORIENTED_EDGE('',*,*,#8834,.T.);
#12083=ORIENTED_EDGE('',*,*,#8835,.F.);
#12084=ORIENTED_EDGE('',*,*,#8836,.T.);
#12085=ORIENTED_EDGE('',*,*,#8837,.T.);
#12086=ORIENTED_EDGE('',*,*,#8838,.F.);
#12087=ORIENTED_EDGE('',*,*,#8839,.T.);
#12088=ORIENTED_EDGE('',*,*,#8840,.F.);
#12089=ORIENTED_EDGE('',*,*,#8841,.F.);
#12090=ORIENTED_EDGE('',*,*,#8842,.F.);
#12091=ORIENTED_EDGE('',*,*,#8843,.F.);
#12092=ORIENTED_EDGE('',*,*,#8844,.T.);
#12093=ORIENTED_EDGE('',*,*,#8845,.T.);
#12094=ORIENTED_EDGE('',*,*,#8846,.F.);
#12095=ORIENTED_EDGE('',*,*,#8847,.T.);
#12096=ORIENTED_EDGE('',*,*,#8848,.F.);
#12097=ORIENTED_EDGE('',*,*,#8849,.F.);
#12098=ORIENTED_EDGE('',*,*,#8850,.F.);
#12099=ORIENTED_EDGE('',*,*,#8851,.F.);
#12100=ORIENTED_EDGE('',*,*,#8852,.T.);
#12101=ORIENTED_EDGE('',*,*,#8853,.F.);
#12102=ORIENTED_EDGE('',*,*,#8854,.T.);
#12103=ORIENTED_EDGE('',*,*,#8855,.F.);
#12104=ORIENTED_EDGE('',*,*,#8856,.F.);
#12105=ORIENTED_EDGE('',*,*,#8857,.F.);
#12106=ORIENTED_EDGE('',*,*,#8858,.F.);
#12107=ORIENTED_EDGE('',*,*,#8859,.F.);
#12108=ORIENTED_EDGE('',*,*,#8860,.F.);
#12109=ORIENTED_EDGE('',*,*,#8849,.T.);
#12110=ORIENTED_EDGE('',*,*,#8861,.T.);
#12111=ORIENTED_EDGE('',*,*,#8862,.T.);
#12112=ORIENTED_EDGE('',*,*,#8848,.T.);
#12113=ORIENTED_EDGE('',*,*,#8841,.T.);
#12114=ORIENTED_EDGE('',*,*,#8863,.T.);
#12115=ORIENTED_EDGE('',*,*,#8864,.T.);
#12116=ORIENTED_EDGE('',*,*,#8840,.T.);
#12117=ORIENTED_EDGE('',*,*,#8833,.T.);
#12118=ORIENTED_EDGE('',*,*,#8865,.T.);
#12119=ORIENTED_EDGE('',*,*,#8866,.T.);
#12120=ORIENTED_EDGE('',*,*,#8867,.T.);
#12121=ORIENTED_EDGE('',*,*,#8868,.F.);
#12122=ORIENTED_EDGE('',*,*,#8869,.T.);
#12123=ORIENTED_EDGE('',*,*,#8870,.T.);
#12124=ORIENTED_EDGE('',*,*,#8869,.F.);
#12125=ORIENTED_EDGE('',*,*,#8871,.F.);
#12126=ORIENTED_EDGE('',*,*,#8872,.T.);
#12127=ORIENTED_EDGE('',*,*,#8873,.T.);
#12128=ORIENTED_EDGE('',*,*,#8872,.F.);
#12129=ORIENTED_EDGE('',*,*,#8874,.T.);
#12130=ORIENTED_EDGE('',*,*,#8875,.T.);
#12131=ORIENTED_EDGE('',*,*,#8876,.T.);
#12132=ORIENTED_EDGE('',*,*,#8877,.T.);
#12133=ORIENTED_EDGE('',*,*,#8878,.T.);
#12134=ORIENTED_EDGE('',*,*,#8879,.T.);
#12135=ORIENTED_EDGE('',*,*,#8880,.T.);
#12136=ORIENTED_EDGE('',*,*,#8826,.T.);
#12137=ORIENTED_EDGE('',*,*,#8881,.T.);
#12138=ORIENTED_EDGE('',*,*,#8858,.T.);
#12139=ORIENTED_EDGE('',*,*,#8882,.T.);
#12140=ORIENTED_EDGE('',*,*,#8846,.T.);
#12141=ORIENTED_EDGE('',*,*,#8883,.T.);
#12142=ORIENTED_EDGE('',*,*,#8884,.T.);
#12143=ORIENTED_EDGE('',*,*,#8885,.T.);
#12144=ORIENTED_EDGE('',*,*,#8838,.T.);
#12145=ORIENTED_EDGE('',*,*,#8886,.T.);
#12146=ORIENTED_EDGE('',*,*,#8887,.T.);
#12147=ORIENTED_EDGE('',*,*,#8888,.T.);
#12148=ORIENTED_EDGE('',*,*,#8889,.T.);
#12149=ORIENTED_EDGE('',*,*,#8890,.F.);
#12150=ORIENTED_EDGE('',*,*,#8891,.T.);
#12151=ORIENTED_EDGE('',*,*,#8878,.F.);
#12152=ORIENTED_EDGE('',*,*,#8892,.T.);
#12153=ORIENTED_EDGE('',*,*,#8893,.F.);
#12154=ORIENTED_EDGE('',*,*,#8894,.T.);
#12155=ORIENTED_EDGE('',*,*,#8874,.F.);
#12156=ORIENTED_EDGE('',*,*,#8895,.T.);
#12157=ORIENTED_EDGE('',*,*,#8882,.F.);
#12158=ORIENTED_EDGE('',*,*,#8896,.T.);
#12159=ORIENTED_EDGE('',*,*,#8897,.F.);
#12160=ORIENTED_EDGE('',*,*,#8898,.T.);
#12161=ORIENTED_EDGE('',*,*,#8885,.F.);
#12162=ORIENTED_EDGE('',*,*,#8899,.T.);
#12163=ORIENTED_EDGE('',*,*,#8900,.F.);
#12164=ORIENTED_EDGE('',*,*,#8901,.T.);
#12165=ORIENTED_EDGE('',*,*,#8902,.F.);
#12166=ORIENTED_EDGE('',*,*,#8903,.T.);
#12167=ORIENTED_EDGE('',*,*,#8904,.F.);
#12168=ORIENTED_EDGE('',*,*,#8905,.T.);
#12169=ORIENTED_EDGE('',*,*,#8880,.F.);
#12170=ORIENTED_EDGE('',*,*,#8906,.T.);
#12171=ORIENTED_EDGE('',*,*,#8907,.F.);
#12172=ORIENTED_EDGE('',*,*,#8908,.T.);
#12173=ORIENTED_EDGE('',*,*,#8876,.F.);
#12174=ORIENTED_EDGE('',*,*,#8909,.T.);
#12175=ORIENTED_EDGE('',*,*,#8910,.F.);
#12176=ORIENTED_EDGE('',*,*,#8911,.T.);
#12177=ORIENTED_EDGE('',*,*,#8912,.F.);
#12178=ORIENTED_EDGE('',*,*,#8913,.T.);
#12179=ORIENTED_EDGE('',*,*,#8881,.F.);
#12180=ORIENTED_EDGE('',*,*,#8914,.T.);
#12181=ORIENTED_EDGE('',*,*,#8915,.F.);
#12182=ORIENTED_EDGE('',*,*,#8916,.T.);
#12183=ORIENTED_EDGE('',*,*,#8883,.F.);
#12184=ORIENTED_EDGE('',*,*,#8917,.T.);
#12185=ORIENTED_EDGE('',*,*,#8918,.F.);
#12186=ORIENTED_EDGE('',*,*,#8919,.T.);
#12187=ORIENTED_EDGE('',*,*,#8920,.F.);
#12188=ORIENTED_EDGE('',*,*,#8921,.T.);
#12189=ORIENTED_EDGE('',*,*,#8897,.T.);
#12190=ORIENTED_EDGE('',*,*,#8922,.T.);
#12191=ORIENTED_EDGE('',*,*,#8890,.T.);
#12192=ORIENTED_EDGE('',*,*,#8923,.T.);
#12193=ORIENTED_EDGE('',*,*,#8893,.T.);
#12194=ORIENTED_EDGE('',*,*,#8924,.T.);
#12195=ORIENTED_EDGE('',*,*,#8904,.T.);
#12196=ORIENTED_EDGE('',*,*,#8835,.T.);
#12197=ORIENTED_EDGE('',*,*,#8925,.T.);
#12198=ORIENTED_EDGE('',*,*,#8843,.T.);
#12199=ORIENTED_EDGE('',*,*,#8900,.T.);
#12200=ORIENTED_EDGE('',*,*,#8851,.T.);
#12201=ORIENTED_EDGE('',*,*,#8920,.T.);
#12202=ORIENTED_EDGE('',*,*,#8926,.T.);
#12203=ORIENTED_EDGE('',*,*,#8902,.T.);
#12204=ORIENTED_EDGE('',*,*,#8927,.T.);
#12205=ORIENTED_EDGE('',*,*,#8907,.T.);
#12206=ORIENTED_EDGE('',*,*,#8855,.T.);
#12207=ORIENTED_EDGE('',*,*,#8912,.T.);
#12208=ORIENTED_EDGE('',*,*,#8928,.T.);
#12209=ORIENTED_EDGE('',*,*,#8915,.T.);
#12210=ORIENTED_EDGE('',*,*,#8929,.T.);
#12211=ORIENTED_EDGE('',*,*,#8930,.T.);
#12212=ORIENTED_EDGE('',*,*,#8931,.T.);
#12213=ORIENTED_EDGE('',*,*,#8918,.T.);
#12214=ORIENTED_EDGE('',*,*,#8823,.T.);
#12215=ORIENTED_EDGE('',*,*,#8910,.T.);
#12216=ORIENTED_EDGE('',*,*,#8831,.T.);
#12217=ORIENTED_EDGE('',*,*,#8871,.T.);
#12218=ORIENTED_EDGE('',*,*,#8873,.F.);
#12219=ORIENTED_EDGE('',*,*,#8868,.T.);
#12220=ORIENTED_EDGE('',*,*,#8870,.F.);
#12221=ORIENTED_EDGE('',*,*,#8888,.F.);
#12222=ORIENTED_EDGE('',*,*,#8932,.T.);
#12223=ORIENTED_EDGE('',*,*,#8925,.F.);
#12224=ORIENTED_EDGE('',*,*,#8933,.T.);
#12225=ORIENTED_EDGE('',*,*,#8930,.F.);
#12226=ORIENTED_EDGE('',*,*,#8934,.T.);
#12227=ORIENTED_EDGE('',*,*,#8886,.F.);
#12228=ORIENTED_EDGE('',*,*,#8935,.T.);
#12229=ORIENTED_EDGE('',*,*,#8936,.T.);
#12230=ORIENTED_EDGE('',*,*,#8937,.T.);
#12231=ORIENTED_EDGE('',*,*,#8938,.T.);
#12232=ORIENTED_EDGE('',*,*,#8821,.T.);
#12233=ORIENTED_EDGE('',*,*,#8853,.T.);
#12234=ORIENTED_EDGE('',*,*,#8939,.T.);
#12235=ORIENTED_EDGE('',*,*,#8940,.T.);
#12236=ORIENTED_EDGE('',*,*,#8860,.T.);
#12237=ORIENTED_EDGE('',*,*,#8941,.T.);
#12238=ORIENTED_EDGE('',*,*,#8942,.T.);
#12239=ORIENTED_EDGE('',*,*,#8828,.T.);
#12240=ORIENTED_EDGE('',*,*,#8829,.T.);
#12241=ORIENTED_EDGE('',*,*,#8896,.F.);
#12242=ORIENTED_EDGE('',*,*,#8857,.T.);
#12243=ORIENTED_EDGE('',*,*,#8943,.F.);
#12244=ORIENTED_EDGE('',*,*,#8859,.T.);
#12245=ORIENTED_EDGE('',*,*,#8913,.F.);
#12246=ORIENTED_EDGE('',*,*,#8854,.F.);
#12247=ORIENTED_EDGE('',*,*,#8943,.T.);
#12248=ORIENTED_EDGE('',*,*,#8940,.F.);
#12249=ORIENTED_EDGE('',*,*,#8944,.F.);
#12250=ORIENTED_EDGE('',*,*,#8922,.F.);
#12251=ORIENTED_EDGE('',*,*,#8891,.F.);
#12252=ORIENTED_EDGE('',*,*,#8944,.T.);
#12253=ORIENTED_EDGE('',*,*,#8945,.F.);
#12254=ORIENTED_EDGE('',*,*,#8856,.T.);
#12255=ORIENTED_EDGE('',*,*,#8906,.F.);
#12256=ORIENTED_EDGE('',*,*,#8946,.F.);
#12257=ORIENTED_EDGE('',*,*,#8945,.T.);
#12258=ORIENTED_EDGE('',*,*,#8939,.F.);
#12259=ORIENTED_EDGE('',*,*,#8946,.T.);
#12260=ORIENTED_EDGE('',*,*,#8879,.F.);
#12261=ORIENTED_EDGE('',*,*,#8947,.F.);
#12262=ORIENTED_EDGE('',*,*,#8884,.F.);
#12263=ORIENTED_EDGE('',*,*,#8948,.F.);
#12264=ORIENTED_EDGE('',*,*,#8861,.F.);
#12265=ORIENTED_EDGE('',*,*,#8899,.F.);
#12266=ORIENTED_EDGE('',*,*,#8947,.T.);
#12267=ORIENTED_EDGE('',*,*,#8852,.F.);
#12268=ORIENTED_EDGE('',*,*,#8948,.T.);
#12269=ORIENTED_EDGE('',*,*,#8916,.F.);
#12270=ORIENTED_EDGE('',*,*,#8949,.F.);
#12271=ORIENTED_EDGE('',*,*,#8949,.T.);
#12272=ORIENTED_EDGE('',*,*,#8928,.F.);
#12273=ORIENTED_EDGE('',*,*,#8950,.F.);
#12274=ORIENTED_EDGE('',*,*,#8862,.F.);
#12275=ORIENTED_EDGE('',*,*,#8898,.F.);
#12276=ORIENTED_EDGE('',*,*,#8850,.T.);
#12277=ORIENTED_EDGE('',*,*,#8847,.F.);
#12278=ORIENTED_EDGE('',*,*,#8950,.T.);
#12279=ORIENTED_EDGE('',*,*,#8914,.F.);
#12280=ORIENTED_EDGE('',*,*,#8845,.F.);
#12281=ORIENTED_EDGE('',*,*,#8951,.F.);
#12282=ORIENTED_EDGE('',*,*,#8887,.F.);
#12283=ORIENTED_EDGE('',*,*,#8952,.F.);
#12284=ORIENTED_EDGE('',*,*,#8863,.F.);
#12285=ORIENTED_EDGE('',*,*,#8932,.F.);
#12286=ORIENTED_EDGE('',*,*,#8951,.T.);
#12287=ORIENTED_EDGE('',*,*,#8844,.F.);
#12288=ORIENTED_EDGE('',*,*,#8952,.T.);
#12289=ORIENTED_EDGE('',*,*,#8934,.F.);
#12290=ORIENTED_EDGE('',*,*,#8953,.F.);
#12291=ORIENTED_EDGE('',*,*,#8953,.T.);
#12292=ORIENTED_EDGE('',*,*,#8929,.F.);
#12293=ORIENTED_EDGE('',*,*,#8954,.F.);
#12294=ORIENTED_EDGE('',*,*,#8864,.F.);
#12295=ORIENTED_EDGE('',*,*,#8901,.F.);
#12296=ORIENTED_EDGE('',*,*,#8842,.T.);
#12297=ORIENTED_EDGE('',*,*,#8839,.F.);
#12298=ORIENTED_EDGE('',*,*,#8954,.T.);
#12299=ORIENTED_EDGE('',*,*,#8917,.F.);
#12300=ORIENTED_EDGE('',*,*,#8837,.F.);
#12301=ORIENTED_EDGE('',*,*,#8955,.F.);
#12302=ORIENTED_EDGE('',*,*,#8931,.F.);
#12303=ORIENTED_EDGE('',*,*,#8956,.F.);
#12304=ORIENTED_EDGE('',*,*,#8866,.F.);
#12305=ORIENTED_EDGE('',*,*,#8919,.F.);
#12306=ORIENTED_EDGE('',*,*,#8955,.T.);
#12307=ORIENTED_EDGE('',*,*,#8957,.F.);
#12308=ORIENTED_EDGE('',*,*,#8956,.T.);
#12309=ORIENTED_EDGE('',*,*,#8935,.F.);
#12310=ORIENTED_EDGE('',*,*,#8958,.F.);
#12311=ORIENTED_EDGE('',*,*,#8957,.T.);
#12312=ORIENTED_EDGE('',*,*,#8865,.F.);
#12313=ORIENTED_EDGE('',*,*,#8959,.F.);
#12314=ORIENTED_EDGE('',*,*,#8926,.F.);
#12315=ORIENTED_EDGE('',*,*,#8958,.T.);
#12316=ORIENTED_EDGE('',*,*,#8889,.F.);
#12317=ORIENTED_EDGE('',*,*,#8960,.F.);
#12318=ORIENTED_EDGE('',*,*,#8867,.F.);
#12319=ORIENTED_EDGE('',*,*,#8903,.F.);
#12320=ORIENTED_EDGE('',*,*,#8959,.T.);
#12321=ORIENTED_EDGE('',*,*,#8836,.F.);
#12322=ORIENTED_EDGE('',*,*,#8960,.T.);
#12323=ORIENTED_EDGE('',*,*,#8933,.F.);
#12324=ORIENTED_EDGE('',*,*,#8834,.F.);
#12325=ORIENTED_EDGE('',*,*,#8908,.F.);
#12326=ORIENTED_EDGE('',*,*,#8830,.T.);
#12327=ORIENTED_EDGE('',*,*,#8827,.F.);
#12328=ORIENTED_EDGE('',*,*,#8832,.T.);
#12329=ORIENTED_EDGE('',*,*,#8909,.F.);
#12330=ORIENTED_EDGE('',*,*,#8961,.F.);
#12331=ORIENTED_EDGE('',*,*,#8961,.T.);
#12332=ORIENTED_EDGE('',*,*,#8875,.F.);
#12333=ORIENTED_EDGE('',*,*,#8962,.F.);
#12334=ORIENTED_EDGE('',*,*,#8941,.F.);
#12335=ORIENTED_EDGE('',*,*,#8892,.F.);
#12336=ORIENTED_EDGE('',*,*,#8825,.T.);
#12337=ORIENTED_EDGE('',*,*,#8963,.F.);
#12338=ORIENTED_EDGE('',*,*,#8962,.T.);
#12339=ORIENTED_EDGE('',*,*,#8894,.F.);
#12340=ORIENTED_EDGE('',*,*,#8964,.F.);
#12341=ORIENTED_EDGE('',*,*,#8963,.T.);
#12342=ORIENTED_EDGE('',*,*,#8942,.F.);
#12343=ORIENTED_EDGE('',*,*,#8964,.T.);
#12344=ORIENTED_EDGE('',*,*,#8923,.F.);
#12345=ORIENTED_EDGE('',*,*,#8911,.F.);
#12346=ORIENTED_EDGE('',*,*,#8822,.T.);
#12347=ORIENTED_EDGE('',*,*,#8965,.F.);
#12348=ORIENTED_EDGE('',*,*,#8824,.T.);
#12349=ORIENTED_EDGE('',*,*,#8921,.F.);
#12350=ORIENTED_EDGE('',*,*,#8966,.F.);
#12351=ORIENTED_EDGE('',*,*,#8965,.T.);
#12352=ORIENTED_EDGE('',*,*,#8938,.F.);
#12353=ORIENTED_EDGE('',*,*,#8967,.F.);
#12354=ORIENTED_EDGE('',*,*,#8877,.F.);
#12355=ORIENTED_EDGE('',*,*,#8966,.T.);
#12356=ORIENTED_EDGE('',*,*,#8927,.F.);
#12357=ORIENTED_EDGE('',*,*,#8968,.F.);
#12358=ORIENTED_EDGE('',*,*,#8936,.F.);
#12359=ORIENTED_EDGE('',*,*,#8895,.F.);
#12360=ORIENTED_EDGE('',*,*,#8967,.T.);
#12361=ORIENTED_EDGE('',*,*,#8969,.F.);
#12362=ORIENTED_EDGE('',*,*,#8968,.T.);
#12363=ORIENTED_EDGE('',*,*,#8905,.F.);
#12364=ORIENTED_EDGE('',*,*,#8970,.F.);
#12365=ORIENTED_EDGE('',*,*,#8969,.T.);
#12366=ORIENTED_EDGE('',*,*,#8937,.F.);
#12367=ORIENTED_EDGE('',*,*,#8970,.T.);
#12368=ORIENTED_EDGE('',*,*,#8924,.F.);
#16349=CYLINDRICAL_SURFACE('',#18250,2.);
#16350=CYLINDRICAL_SURFACE('',#18263,2.);
#16351=CYLINDRICAL_SURFACE('',#18271,2.);
#16352=CYLINDRICAL_SURFACE('',#18284,2.);
#16353=CYLINDRICAL_SURFACE('',#18287,6.00000000000143);
#16354=CYLINDRICAL_SURFACE('',#18289,6.00000000000152);
#16355=CYLINDRICAL_SURFACE('',#18291,6.00000000000095);
#16356=CYLINDRICAL_SURFACE('',#18293,5.);
#16357=CYLINDRICAL_SURFACE('',#18296,12.5);
#16358=CYLINDRICAL_SURFACE('',#18299,25.);
#16359=CYLINDRICAL_SURFACE('',#18302,25.);
#16360=CYLINDRICAL_SURFACE('',#18305,25.);
#16361=CYLINDRICAL_SURFACE('',#18308,25.);
#16362=CYLINDRICAL_SURFACE('',#18311,25.);
#16363=CYLINDRICAL_SURFACE('',#18361,25.);
#16364=CYLINDRICAL_SURFACE('',#18375,6.00000000000022);
#16365=CYLINDRICAL_SURFACE('',#18377,6.00000000000081);
#16366=CYLINDRICAL_SURFACE('',#18379,6.);
#16367=CYLINDRICAL_SURFACE('',#18390,2.);
#16368=CYLINDRICAL_SURFACE('',#18391,2.);
#16369=CYLINDRICAL_SURFACE('',#18401,2.);
#16370=CYLINDRICAL_SURFACE('',#18418,2.);
#16371=CYLINDRICAL_SURFACE('',#18420,2.);
#16372=CYLINDRICAL_SURFACE('',#18427,2.);
#16373=CYLINDRICAL_SURFACE('',#18438,2.);
#16374=CYLINDRICAL_SURFACE('',#18440,2.);
#16850=ADVANCED_FACE('',(#1891),#155,.T.);
#16851=ADVANCED_FACE('',(#1892),#16349,.T.);
#16852=ADVANCED_FACE('',(#1893),#156,.T.);
#16853=ADVANCED_FACE('',(#1894),#157,.T.);
#16854=ADVANCED_FACE('',(#1895),#16350,.T.);
#16855=ADVANCED_FACE('',(#1896),#158,.T.);
#16856=ADVANCED_FACE('',(#1897),#16351,.T.);
#16857=ADVANCED_FACE('',(#1898),#159,.T.);
#16858=ADVANCED_FACE('',(#1899),#160,.T.);
#16859=ADVANCED_FACE('',(#1900),#16352,.T.);
#16860=ADVANCED_FACE('',(#1901),#16353,.F.);
#16861=ADVANCED_FACE('',(#1902),#16354,.F.);
#16862=ADVANCED_FACE('',(#1903),#16355,.F.);
#16863=ADVANCED_FACE('',(#1904),#16356,.F.);
#16864=ADVANCED_FACE('',(#1905),#16357,.T.);
#16865=ADVANCED_FACE('',(#1906),#16358,.T.);
#16866=ADVANCED_FACE('',(#1907),#16359,.T.);
#16867=ADVANCED_FACE('',(#1908),#16360,.T.);
#16868=ADVANCED_FACE('',(#1909),#16361,.T.);
#16869=ADVANCED_FACE('',(#1910),#16362,.T.);
#16870=ADVANCED_FACE('',(#1911),#161,.T.);
#16871=ADVANCED_FACE('',(#1912),#162,.T.);
#16872=ADVANCED_FACE('',(#1913),#163,.T.);
#16873=ADVANCED_FACE('',(#1914),#164,.T.);
#16874=ADVANCED_FACE('',(#1915),#165,.T.);
#16875=ADVANCED_FACE('',(#1916),#166,.T.);
#16876=ADVANCED_FACE('',(#1917),#167,.T.);
#16877=ADVANCED_FACE('',(#1918),#168,.T.);
#16878=ADVANCED_FACE('',(#1919),#169,.T.);
#16879=ADVANCED_FACE('',(#1920),#170,.T.);
#16880=ADVANCED_FACE('',(#1921),#1275,.F.);
#16881=ADVANCED_FACE('',(#1922),#16363,.T.);
#16882=ADVANCED_FACE('',(#1923,#883),#1276,.F.);
#16883=ADVANCED_FACE('',(#1924,#884),#1277,.F.);
#16884=ADVANCED_FACE('',(#1925),#1278,.F.);
#16885=ADVANCED_FACE('',(#1926),#171,.T.);
#16886=ADVANCED_FACE('',(#1927),#172,.T.);
#16887=ADVANCED_FACE('',(#1928),#16364,.F.);
#16888=ADVANCED_FACE('',(#1929),#16365,.F.);
#16889=ADVANCED_FACE('',(#1930),#16366,.F.);
#16890=ADVANCED_FACE('',(#1931),#93,.T.);
#16891=ADVANCED_FACE('',(#1932),#94,.T.);
#16892=ADVANCED_FACE('',(#1933),#173,.T.);
#16893=ADVANCED_FACE('',(#1934),#95,.T.);
#16894=ADVANCED_FACE('',(#1935),#96,.T.);
#16895=ADVANCED_FACE('',(#1936),#16367,.T.);
#16896=ADVANCED_FACE('',(#1937),#16368,.T.);
#16897=ADVANCED_FACE('',(#1938),#97,.T.);
#16898=ADVANCED_FACE('',(#1939),#98,.T.);
#16899=ADVANCED_FACE('',(#1940),#174,.T.);
#16900=ADVANCED_FACE('',(#1941),#99,.T.);
#16901=ADVANCED_FACE('',(#1942),#100,.T.);
#16902=ADVANCED_FACE('',(#1943),#16369,.T.);
#16903=ADVANCED_FACE('',(#1944),#101,.T.);
#16904=ADVANCED_FACE('',(#1945),#102,.T.);
#16905=ADVANCED_FACE('',(#1946),#175,.T.);
#16906=ADVANCED_FACE('',(#1947),#103,.T.);
#16907=ADVANCED_FACE('',(#1948),#104,.T.);
#16908=ADVANCED_FACE('',(#1949),#176,.T.);
#16909=ADVANCED_FACE('',(#1950),#105,.T.);
#16910=ADVANCED_FACE('',(#1951),#106,.T.);
#16911=ADVANCED_FACE('',(#1952),#16370,.T.);
#16912=ADVANCED_FACE('',(#1953),#16371,.T.);
#16913=ADVANCED_FACE('',(#1954),#107,.T.);
#16914=ADVANCED_FACE('',(#1955),#108,.T.);
#16915=ADVANCED_FACE('',(#1956),#109,.T.);
#16916=ADVANCED_FACE('',(#1957),#110,.T.);
#16917=ADVANCED_FACE('',(#1958),#16372,.T.);
#16918=ADVANCED_FACE('',(#1959),#111,.T.);
#16919=ADVANCED_FACE('',(#1960),#112,.T.);
#16920=ADVANCED_FACE('',(#1961),#177,.T.);
#16921=ADVANCED_FACE('',(#1962),#113,.T.);
#16922=ADVANCED_FACE('',(#1963),#114,.T.);
#16923=ADVANCED_FACE('',(#1964),#16373,.T.);
#16924=ADVANCED_FACE('',(#1965),#16374,.T.);
#16925=ADVANCED_FACE('',(#1966),#115,.T.);
#16926=ADVANCED_FACE('',(#1967),#116,.T.);
#16927=ADVANCED_FACE('',(#1968),#178,.T.);
#17624=CLOSED_SHELL('',(#16850,#16851,#16852,#16853,#16854,#16855,#16856,
#16857,#16858,#16859,#16860,#16861,#16862,#16863,#16864,#16865,#16866,#16867,
#16868,#16869,#16870,#16871,#16872,#16873,#16874,#16875,#16876,#16877,#16878,
#16879,#16880,#16881,#16882,#16883,#16884,#16885,#16886,#16887,#16888,#16889,
#16890,#16891,#16892,#16893,#16894,#16895,#16896,#16897,#16898,#16899,#16900,
#16901,#16902,#16903,#16904,#16905,#16906,#16907,#16908,#16909,#16910,#16911,
#16912,#16913,#16914,#16915,#16916,#16917,#16918,#16919,#16920,#16921,#16922,
#16923,#16924,#16925,#16926,#16927));
#18244=AXIS2_PLACEMENT_3D('',#33054,#20877,#20878);
#18245=AXIS2_PLACEMENT_3D('',#33055,#20879,#20880);
#18246=AXIS2_PLACEMENT_3D('',#33058,#20881,#20882);
#18247=AXIS2_PLACEMENT_3D('',#33060,#20883,#20884);
#18248=AXIS2_PLACEMENT_3D('',#33062,#20885,#20886);
#18249=AXIS2_PLACEMENT_3D('',#33063,#20887,#20888);
#18250=AXIS2_PLACEMENT_3D('',#33064,#20889,#20890);
#18251=AXIS2_PLACEMENT_3D('',#33067,#20891,#20892);
#18252=AXIS2_PLACEMENT_3D('',#33071,#20894,#20895);
#18253=AXIS2_PLACEMENT_3D('',#33073,#20897,#20898);
#18254=AXIS2_PLACEMENT_3D('',#33075,#20899,#20900);
#18255=AXIS2_PLACEMENT_3D('',#33077,#20901,#20902);
#18256=AXIS2_PLACEMENT_3D('',#33079,#20903,#20904);
#18257=AXIS2_PLACEMENT_3D('',#33080,#20905,#20906);
#18258=AXIS2_PLACEMENT_3D('',#33081,#20907,#20908);
#18259=AXIS2_PLACEMENT_3D('',#33084,#20909,#20910);
#18260=AXIS2_PLACEMENT_3D('',#33086,#20911,#20912);
#18261=AXIS2_PLACEMENT_3D('',#33088,#20913,#20914);
#18262=AXIS2_PLACEMENT_3D('',#33089,#20915,#20916);
#18263=AXIS2_PLACEMENT_3D('',#33090,#20917,#20918);
#18264=AXIS2_PLACEMENT_3D('',#33093,#20919,#20920);
#18265=AXIS2_PLACEMENT_3D('',#33097,#20922,#20923);
#18266=AXIS2_PLACEMENT_3D('',#33099,#20925,#20926);
#18267=AXIS2_PLACEMENT_3D('',#33101,#20927,#20928);
#18268=AXIS2_PLACEMENT_3D('',#33103,#20929,#20930);
#18269=AXIS2_PLACEMENT_3D('',#33105,#20931,#20932);
#18270=AXIS2_PLACEMENT_3D('',#33106,#20933,#20934);
#18271=AXIS2_PLACEMENT_3D('',#33107,#20935,#20936);
#18272=AXIS2_PLACEMENT_3D('',#33110,#20937,#20938);
#18273=AXIS2_PLACEMENT_3D('',#33114,#20940,#20941);
#18274=AXIS2_PLACEMENT_3D('',#33116,#20943,#20944);
#18275=AXIS2_PLACEMENT_3D('',#33118,#20945,#20946);
#18276=AXIS2_PLACEMENT_3D('',#33120,#20947,#20948);
#18277=AXIS2_PLACEMENT_3D('',#33122,#20949,#20950);
#18278=AXIS2_PLACEMENT_3D('',#33123,#20951,#20952);
#18279=AXIS2_PLACEMENT_3D('',#33124,#20953,#20954);
#18280=AXIS2_PLACEMENT_3D('',#33127,#20955,#20956);
#18281=AXIS2_PLACEMENT_3D('',#33129,#20957,#20958);
#18282=AXIS2_PLACEMENT_3D('',#33131,#20959,#20960);
#18283=AXIS2_PLACEMENT_3D('',#33132,#20961,#20962);
#18284=AXIS2_PLACEMENT_3D('',#33133,#20963,#20964);
#18285=AXIS2_PLACEMENT_3D('',#33136,#20965,#20966);
#18286=AXIS2_PLACEMENT_3D('',#33139,#20968,#20969);
#18287=AXIS2_PLACEMENT_3D('',#33141,#20971,#20972);
#18288=AXIS2_PLACEMENT_3D('',#33144,#20974,#20975);
#18289=AXIS2_PLACEMENT_3D('',#33145,#20976,#20977);
#18290=AXIS2_PLACEMENT_3D('',#33148,#20979,#20980);
#18291=AXIS2_PLACEMENT_3D('',#33149,#20981,#20982);
#18292=AXIS2_PLACEMENT_3D('',#33153,#20984,#20985);
#18293=AXIS2_PLACEMENT_3D('',#33155,#20987,#20988);
#18294=AXIS2_PLACEMENT_3D('',#33157,#20989,#20990);
#18295=AXIS2_PLACEMENT_3D('',#33160,#20992,#20993);
#18296=AXIS2_PLACEMENT_3D('',#33161,#20994,#20995);
#18297=AXIS2_PLACEMENT_3D('',#33163,#20996,#20997);
#18298=AXIS2_PLACEMENT_3D('',#33166,#20999,#21000);
#18299=AXIS2_PLACEMENT_3D('',#33167,#21001,#21002);
#18300=AXIS2_PLACEMENT_3D('',#33170,#21003,#21004);
#18301=AXIS2_PLACEMENT_3D('',#33174,#21006,#21007);
#18302=AXIS2_PLACEMENT_3D('',#33176,#21009,#21010);
#18303=AXIS2_PLACEMENT_3D('',#33178,#21011,#21012);
#18304=AXIS2_PLACEMENT_3D('',#33181,#21014,#21015);
#18305=AXIS2_PLACEMENT_3D('',#33182,#21016,#21017);
#18306=AXIS2_PLACEMENT_3D('',#33183,#21018,#21019);
#18307=AXIS2_PLACEMENT_3D('',#33184,#21020,#21021);
#18308=AXIS2_PLACEMENT_3D('',#33185,#21022,#21023);
#18309=AXIS2_PLACEMENT_3D('',#33187,#21024,#21025);
#18310=AXIS2_PLACEMENT_3D('',#33190,#21027,#21028);
#18311=AXIS2_PLACEMENT_3D('',#33191,#21029,#21030);
#18312=AXIS2_PLACEMENT_3D('',#33194,#21031,#21032);
#18313=AXIS2_PLACEMENT_3D('',#33198,#21034,#21035);
#18314=AXIS2_PLACEMENT_3D('',#33200,#21037,#21038);
#18315=AXIS2_PLACEMENT_3D('',#33203,#21039,#21040);
#18316=AXIS2_PLACEMENT_3D('',#33204,#21041,#21042);
#18317=AXIS2_PLACEMENT_3D('',#33205,#21043,#21044);
#18318=AXIS2_PLACEMENT_3D('',#33206,#21045,#21046);
#18319=AXIS2_PLACEMENT_3D('',#33209,#21047,#21048);
#18320=AXIS2_PLACEMENT_3D('',#33210,#21049,#21050);
#18321=AXIS2_PLACEMENT_3D('',#33211,#21051,#21052);
#18322=AXIS2_PLACEMENT_3D('',#33212,#21053,#21054);
#18323=AXIS2_PLACEMENT_3D('',#33214,#21055,#21056);
#18324=AXIS2_PLACEMENT_3D('',#33215,#21057,#21058);
#18325=AXIS2_PLACEMENT_3D('',#33216,#21059,#21060);
#18326=AXIS2_PLACEMENT_3D('',#33217,#21061,#21062);
#18327=AXIS2_PLACEMENT_3D('',#33218,#21063,#21064);
#18328=AXIS2_PLACEMENT_3D('',#33219,#21065,#21066);
#18329=AXIS2_PLACEMENT_3D('',#33220,#21067,#21068);
#18330=AXIS2_PLACEMENT_3D('',#33221,#21069,#21070);
#18331=AXIS2_PLACEMENT_3D('',#33224,#21071,#21072);
#18332=AXIS2_PLACEMENT_3D('',#33225,#21073,#21074);
#18333=AXIS2_PLACEMENT_3D('',#33227,#21075,#21076);
#18334=AXIS2_PLACEMENT_3D('',#33228,#21077,#21078);
#18335=AXIS2_PLACEMENT_3D('',#33229,#21079,#21080);
#18336=AXIS2_PLACEMENT_3D('',#33230,#21081,#21082);
#18337=AXIS2_PLACEMENT_3D('',#33231,#21083,#21084);
#18338=AXIS2_PLACEMENT_3D('',#33232,#21085,#21086);
#18339=AXIS2_PLACEMENT_3D('',#33233,#21087,#21088);
#18340=AXIS2_PLACEMENT_3D('',#33234,#21089,#21090);
#18341=AXIS2_PLACEMENT_3D('',#33235,#21091,#21092);
#18342=AXIS2_PLACEMENT_3D('',#33236,#21093,#21094);
#18343=AXIS2_PLACEMENT_3D('',#33237,#21095,#21096);
#18344=AXIS2_PLACEMENT_3D('',#33239,#21097,#21098);
#18345=AXIS2_PLACEMENT_3D('',#33240,#21099,#21100);
#18346=AXIS2_PLACEMENT_3D('',#33241,#21101,#21102);
#18347=AXIS2_PLACEMENT_3D('',#33242,#21103,#21104);
#18348=AXIS2_PLACEMENT_3D('',#33245,#21105,#21106);
#18349=AXIS2_PLACEMENT_3D('',#33246,#21107,#21108);
#18350=AXIS2_PLACEMENT_3D('',#33247,#21109,#21110);
#18351=AXIS2_PLACEMENT_3D('',#33248,#21111,#21112);
#18352=AXIS2_PLACEMENT_3D('',#33250,#21113,#21114);
#18353=AXIS2_PLACEMENT_3D('',#33252,#21115,#21116);
#18354=AXIS2_PLACEMENT_3D('',#33254,#21117,#21118);
#18355=AXIS2_PLACEMENT_3D('',#33255,#21119,#21120);
#18356=AXIS2_PLACEMENT_3D('',#33256,#21121,#21122);
#18357=AXIS2_PLACEMENT_3D('',#33257,#21123,#21124);
#18358=AXIS2_PLACEMENT_3D('',#33258,#21125,#21126);
#18359=AXIS2_PLACEMENT_3D('',#33259,#21127,#21128);
#18360=AXIS2_PLACEMENT_3D('',#33260,#21129,#21130);
#18361=AXIS2_PLACEMENT_3D('',#33261,#21131,#21132);
#18362=AXIS2_PLACEMENT_3D('',#33264,#21135,#21136);
#18363=AXIS2_PLACEMENT_3D('',#33265,#21137,#21138);
#18364=AXIS2_PLACEMENT_3D('',#33267,#21139,#21140);
#18365=AXIS2_PLACEMENT_3D('',#33269,#21141,#21142);
#18366=AXIS2_PLACEMENT_3D('',#33270,#21143,#21144);
#18367=AXIS2_PLACEMENT_3D('',#33271,#21145,#21146);
#18368=AXIS2_PLACEMENT_3D('',#33272,#21147,#21148);
#18369=AXIS2_PLACEMENT_3D('',#33273,#21149,#21150);
#18370=AXIS2_PLACEMENT_3D('',#33274,#21151,#21152);
#18371=AXIS2_PLACEMENT_3D('',#33275,#21153,#21154);
#18372=AXIS2_PLACEMENT_3D('',#33276,#21155,#21156);
#18373=AXIS2_PLACEMENT_3D('',#33277,#21157,#21158);
#18374=AXIS2_PLACEMENT_3D('',#33278,#21159,#21160);
#18375=AXIS2_PLACEMENT_3D('',#33279,#21161,#21162);
#18376=AXIS2_PLACEMENT_3D('',#33283,#21164,#21165);
#18377=AXIS2_PLACEMENT_3D('',#33285,#21167,#21168);
#18378=AXIS2_PLACEMENT_3D('',#33288,#21170,#21171);
#18379=AXIS2_PLACEMENT_3D('',#33289,#21172,#21173);
#18380=AXIS2_PLACEMENT_3D('',#33292,#21175,#21176);
#18381=AXIS2_PLACEMENT_3D('',#33293,#21177,#21178);
#18382=AXIS2_PLACEMENT_3D('',#33294,#21179,#21180);
#18383=AXIS2_PLACEMENT_3D('',#33295,#21181,#21182);
#18384=AXIS2_PLACEMENT_3D('',#33296,#21183,#21184);
#18385=AXIS2_PLACEMENT_3D('',#33297,#21185,#21186);
#18386=AXIS2_PLACEMENT_3D('',#33298,#21187,#21188);
#18387=AXIS2_PLACEMENT_3D('',#33299,#21189,#21190);
#18388=AXIS2_PLACEMENT_3D('',#33300,#21191,#21192);
#18389=AXIS2_PLACEMENT_3D('',#33301,#21193,#21194);
#18390=AXIS2_PLACEMENT_3D('',#33302,#21195,#21196);
#18391=AXIS2_PLACEMENT_3D('',#33303,#21197,#21198);
#18392=AXIS2_PLACEMENT_3D('',#33304,#21199,#21200);
#18393=AXIS2_PLACEMENT_3D('',#33305,#21201,#21202);
#18394=AXIS2_PLACEMENT_3D('',#33306,#21203,#21204);
#18395=AXIS2_PLACEMENT_3D('',#33307,#21205,#21206);
#18396=AXIS2_PLACEMENT_3D('',#33308,#21207,#21208);
#18397=AXIS2_PLACEMENT_3D('',#33309,#21209,#21210);
#18398=AXIS2_PLACEMENT_3D('',#33310,#21211,#21212);
#18399=AXIS2_PLACEMENT_3D('',#33311,#21213,#21214);
#18400=AXIS2_PLACEMENT_3D('',#33312,#21215,#21216);
#18401=AXIS2_PLACEMENT_3D('',#33313,#21217,#21218);
#18402=AXIS2_PLACEMENT_3D('',#33314,#21219,#21220);
#18403=AXIS2_PLACEMENT_3D('',#33315,#21221,#21222);
#18404=AXIS2_PLACEMENT_3D('',#33316,#21223,#21224);
#18405=AXIS2_PLACEMENT_3D('',#33317,#21225,#21226);
#18406=AXIS2_PLACEMENT_3D('',#33318,#21227,#21228);
#18407=AXIS2_PLACEMENT_3D('',#33319,#21229,#21230);
#18408=AXIS2_PLACEMENT_3D('',#33320,#21231,#21232);
#18409=AXIS2_PLACEMENT_3D('',#33321,#21233,#21234);
#18410=AXIS2_PLACEMENT_3D('',#33322,#21235,#21236);
#18411=AXIS2_PLACEMENT_3D('',#33323,#21237,#21238);
#18412=AXIS2_PLACEMENT_3D('',#33324,#21239,#21240);
#18413=AXIS2_PLACEMENT_3D('',#33325,#21241,#21242);
#18414=AXIS2_PLACEMENT_3D('',#33326,#21243,#21244);
#18415=AXIS2_PLACEMENT_3D('',#33327,#21245,#21246);
#18416=AXIS2_PLACEMENT_3D('',#33328,#21247,#21248);
#18417=AXIS2_PLACEMENT_3D('',#33329,#21249,#21250);
#18418=AXIS2_PLACEMENT_3D('',#33330,#21251,#21252);
#18419=AXIS2_PLACEMENT_3D('',#33331,#21253,#21254);
#18420=AXIS2_PLACEMENT_3D('',#33332,#21255,#21256);
#18421=AXIS2_PLACEMENT_3D('',#33333,#21257,#21258);
#18422=AXIS2_PLACEMENT_3D('',#33334,#21259,#21260);
#18423=AXIS2_PLACEMENT_3D('',#33335,#21261,#21262);
#18424=AXIS2_PLACEMENT_3D('',#33336,#21263,#21264);
#18425=AXIS2_PLACEMENT_3D('',#33337,#21265,#21266);
#18426=AXIS2_PLACEMENT_3D('',#33338,#21267,#21268);
#18427=AXIS2_PLACEMENT_3D('',#33339,#21269,#21270);
#18428=AXIS2_PLACEMENT_3D('',#33340,#21271,#21272);
#18429=AXIS2_PLACEMENT_3D('',#33341,#21273,#21274);
#18430=AXIS2_PLACEMENT_3D('',#33342,#21275,#21276);
#18431=AXIS2_PLACEMENT_3D('',#33343,#21277,#21278);
#18432=AXIS2_PLACEMENT_3D('',#33344,#21279,#21280);
#18433=AXIS2_PLACEMENT_3D('',#33345,#21281,#21282);
#18434=AXIS2_PLACEMENT_3D('',#33346,#21283,#21284);
#18435=AXIS2_PLACEMENT_3D('',#33347,#21285,#21286);
#18436=AXIS2_PLACEMENT_3D('',#33348,#21287,#21288);
#18437=AXIS2_PLACEMENT_3D('',#33349,#21289,#21290);
#18438=AXIS2_PLACEMENT_3D('',#33350,#21291,#21292);
#18439=AXIS2_PLACEMENT_3D('',#33351,#21293,#21294);
#18440=AXIS2_PLACEMENT_3D('',#33352,#21295,#21296);
#18441=AXIS2_PLACEMENT_3D('',#33353,#21297,#21298);
#18442=AXIS2_PLACEMENT_3D('',#33354,#21299,#21300);
#18443=AXIS2_PLACEMENT_3D('',#33355,#21301,#21302);
#18444=AXIS2_PLACEMENT_3D('',#33356,#21303,#21304);
#18445=AXIS2_PLACEMENT_3D('',#33357,#21305,#21306);
#18446=AXIS2_PLACEMENT_3D('',#33358,#21307,#21308);
#20877=DIRECTION('axis',(0.,0.,1.));
#20878=DIRECTION('refdir',(1.,0.,0.));
#20879=DIRECTION('center_axis',(-1.,-1.22464679914735E-16,0.));
#20880=DIRECTION('ref_axis',(1.77635683940021E-16,-1.,0.));
#20881=DIRECTION('center_axis',(1.,1.22464679914735E-16,0.));
#20882=DIRECTION('ref_axis',(1.22464679914735E-16,-1.,0.));
#20883=DIRECTION('center_axis',(0.,0.80466773100941,-0.593725393319309));
#20884=DIRECTION('ref_axis',(0.,0.593725393319309,0.80466773100941));
#20885=DIRECTION('center_axis',(-1.,-1.22464679914735E-16,0.));
#20886=DIRECTION('ref_axis',(1.22464679914735E-16,-1.,0.));
#20887=DIRECTION('center_axis',(-1.72383876846542E-15,0.111847407981753,
-0.993725393319383));
#20888=DIRECTION('ref_axis',(1.05814669609279E-32,0.993725393319383,0.111847407981753));
#20889=DIRECTION('center_axis',(1.,1.22464679914735E-16,0.));
#20890=DIRECTION('ref_axis',(-1.22464679914735E-16,1.,0.));
#20891=DIRECTION('center_axis',(-1.,-1.99493199737333E-16,-8.70659703262162E-17));
#20892=DIRECTION('ref_axis',(1.99493199737333E-16,-1.,-1.51035382683587E-33));
#20893=DIRECTION('',(-1.,-1.22464679914735E-16,0.));
#20894=DIRECTION('center_axis',(-1.,0.,0.));
#20895=DIRECTION('ref_axis',(0.,0.,1.));
#20896=DIRECTION('',(1.,1.22464679914735E-16,0.));
#20897=DIRECTION('center_axis',(-1.,-1.22464679914735E-16,0.));
#20898=DIRECTION('ref_axis',(1.77635683940025E-16,-1.,0.));
#20899=DIRECTION('center_axis',(1.,1.22464679914735E-16,0.));
#20900=DIRECTION('ref_axis',(1.22464679914735E-16,-1.,0.));
#20901=DIRECTION('center_axis',(0.,0.916515138991168,0.400000000000001));
#20902=DIRECTION('ref_axis',(0.,-0.400000000000001,0.916515138991168));
#20903=DIRECTION('center_axis',(-1.,-1.22464679914735E-16,0.));
#20904=DIRECTION('ref_axis',(1.22464679914735E-16,-1.,0.));
#20905=DIRECTION('center_axis',(-1.7347234759768E-16,0.916515138991168,
-0.399999999999999));
#20906=DIRECTION('ref_axis',(-1.38807035205952E-32,0.399999999999999,0.916515138991168));
#20907=DIRECTION('center_axis',(1.,1.22464679914735E-16,0.));
#20908=DIRECTION('ref_axis',(-1.33226762955006E-16,1.,0.));
#20909=DIRECTION('center_axis',(-1.,-1.22464679914735E-16,0.));
#20910=DIRECTION('ref_axis',(-1.22464679914735E-16,1.,0.));
#20911=DIRECTION('center_axis',(5.1497468903733E-16,0.804667731009371,0.593725393319361));
#20912=DIRECTION('ref_axis',(-8.01741870322078E-32,-0.593725393319361,0.804667731009371));
#20913=DIRECTION('center_axis',(1.,1.22464679914735E-16,0.));
#20914=DIRECTION('ref_axis',(-1.22464679914735E-16,1.,0.));
#20915=DIRECTION('center_axis',(0.,0.111847407981704,0.993725393319389));
#20916=DIRECTION('ref_axis',(0.,-0.993725393319389,0.111847407981704));
#20917=DIRECTION('center_axis',(-1.,-1.22464679914735E-16,0.));
#20918=DIRECTION('ref_axis',(1.22464679914735E-16,-1.,0.));
#20919=DIRECTION('center_axis',(-1.,0.,0.));
#20920=DIRECTION('ref_axis',(0.,0.,1.));
#20921=DIRECTION('',(1.,1.22464679914735E-16,0.));
#20922=DIRECTION('center_axis',(1.,1.99493199737338E-16,-8.70659703262009E-17));
#20923=DIRECTION('ref_axis',(-1.99493199737338E-16,1.,-1.51035382683516E-33));
#20924=DIRECTION('',(-1.,-1.22464679914735E-16,0.));
#20925=DIRECTION('center_axis',(1.,1.22464679914735E-16,0.));
#20926=DIRECTION('ref_axis',(-1.33226762954999E-16,1.,0.));
#20927=DIRECTION('center_axis',(-1.,-1.22464679914735E-16,0.));
#20928=DIRECTION('ref_axis',(-1.22464679914735E-16,1.,0.));
#20929=DIRECTION('center_axis',(0.,-0.916515138991197,0.399999999999934));
#20930=DIRECTION('ref_axis',(0.,-0.399999999999934,-0.916515138991197));
#20931=DIRECTION('center_axis',(1.,1.22464679914735E-16,0.));
#20932=DIRECTION('ref_axis',(-1.22464679914735E-16,1.,0.));
#20933=DIRECTION('center_axis',(-1.76337267529379E-15,0.916515138991152,
0.400000000000037));
#20934=DIRECTION('ref_axis',(-2.36429138143015E-32,-0.400000000000037,0.916515138991152));
#20935=DIRECTION('center_axis',(-1.,-1.22464679914735E-16,0.));
#20936=DIRECTION('ref_axis',(1.22464679914735E-16,-1.,0.));
#20937=DIRECTION('center_axis',(-1.,0.,0.));
#20938=DIRECTION('ref_axis',(0.,0.,1.));
#20939=DIRECTION('',(1.,1.22464679914735E-16,0.));
#20940=DIRECTION('center_axis',(1.,2.13362867122434E-16,4.30616635022195E-17));
#20941=DIRECTION('ref_axis',(-2.13362867122434E-16,1.,1.49749836094217E-34));
#20942=DIRECTION('',(-1.,-1.22464679914735E-16,0.));
#20943=DIRECTION('center_axis',(1.,1.22464679914735E-16,0.));
#20944=DIRECTION('ref_axis',(-1.33226762955E-16,1.,0.));
#20945=DIRECTION('center_axis',(-1.,-1.22464679914735E-16,0.));
#20946=DIRECTION('ref_axis',(-1.22464679914735E-16,1.,0.));
#20947=DIRECTION('center_axis',(0.,-0.111847407981938,0.993725393319363));
#20948=DIRECTION('ref_axis',(0.,-0.993725393319363,-0.111847407981938));
#20949=DIRECTION('center_axis',(1.,1.22464679914735E-16,0.));
#20950=DIRECTION('ref_axis',(-1.22464679914735E-16,1.,0.));
#20951=DIRECTION('center_axis',(0.,0.804667731009333,-0.593725393319413));
#20952=DIRECTION('ref_axis',(0.,0.593725393319413,0.804667731009333));
#20953=DIRECTION('center_axis',(-1.,-1.22464679914735E-16,0.));
#20954=DIRECTION('ref_axis',(1.77635683940011E-16,-1.,0.));
#20955=DIRECTION('center_axis',(1.,1.22464679914735E-16,0.));
#20956=DIRECTION('ref_axis',(1.22464679914735E-16,-1.,0.));
#20957=DIRECTION('center_axis',(-1.7238387684654E-15,-0.111847407981876,
-0.99372539331937));
#20958=DIRECTION('ref_axis',(-7.80419006320916E-33,0.99372539331937,-0.111847407981876));
#20959=DIRECTION('center_axis',(-1.,-1.22464679914735E-16,0.));
#20960=DIRECTION('ref_axis',(1.22464679914735E-16,-1.,0.));
#20961=DIRECTION('center_axis',(-2.42582538141765E-15,0.804667731009302,
0.593725393319455));
#20962=DIRECTION('ref_axis',(-5.51486489057277E-31,-0.593725393319454,0.804667731009302));
#20963=DIRECTION('center_axis',(1.,1.22464679914735E-16,0.));
#20964=DIRECTION('ref_axis',(-1.22464679914735E-16,1.,0.));
#20965=DIRECTION('center_axis',(-1.,0.,0.));
#20966=DIRECTION('ref_axis',(0.,0.,1.));
#20967=DIRECTION('',(-1.,-1.22464679914735E-16,0.));
#20968=DIRECTION('center_axis',(1.,0.,0.));
#20969=DIRECTION('ref_axis',(0.,0.,-1.));
#20970=DIRECTION('',(1.,1.22464679914735E-16,0.));
#20971=DIRECTION('center_axis',(1.,1.22464679914735E-16,0.));
#20972=DIRECTION('ref_axis',(-1.22464679914735E-16,1.,0.));
#20973=DIRECTION('',(1.,1.22464679914735E-16,0.));
#20974=DIRECTION('center_axis',(1.,1.22464679914735E-16,0.));
#20975=DIRECTION('ref_axis',(1.22464679914735E-16,-1.,0.));
#20976=DIRECTION('center_axis',(1.,1.22464679914735E-16,0.));
#20977=DIRECTION('ref_axis',(-1.22464679914735E-16,1.,0.));
#20978=DIRECTION('',(1.,1.22464679914735E-16,0.));
#20979=DIRECTION('center_axis',(1.,1.22464679914735E-16,0.));
#20980=DIRECTION('ref_axis',(1.22464679914735E-16,-1.,1.77635683940026E-15));
#20981=DIRECTION('center_axis',(1.,1.22464679914735E-16,0.));
#20982=DIRECTION('ref_axis',(-1.22464679914735E-16,1.,0.));
#20983=DIRECTION('',(1.,1.22464679914735E-16,0.));
#20984=DIRECTION('center_axis',(1.,1.22464679914735E-16,0.));
#20985=DIRECTION('ref_axis',(1.22464679914735E-16,-1.,1.15648231731769E-15));
#20986=DIRECTION('',(-1.,-1.22464679914735E-16,0.));
#20987=DIRECTION('center_axis',(-1.,-1.22464679914735E-16,0.));
#20988=DIRECTION('ref_axis',(1.22464679914735E-16,-1.,0.));
#20989=DIRECTION('center_axis',(-1.,-1.22464679914735E-16,0.));
#20990=DIRECTION('ref_axis',(1.22464679914735E-16,-1.,0.));
#20991=DIRECTION('',(-1.,-1.22464679914735E-16,0.));
#20992=DIRECTION('center_axis',(-1.,-1.22464679914735E-16,0.));
#20993=DIRECTION('ref_axis',(1.22464679914735E-16,-1.,0.));
#20994=DIRECTION('center_axis',(-1.,-1.22464679914735E-16,0.));
#20995=DIRECTION('ref_axis',(1.22464679914735E-16,-1.,0.));
#20996=DIRECTION('center_axis',(-1.,-1.22464679914735E-16,0.));
#20997=DIRECTION('ref_axis',(1.22464679914735E-16,-1.,0.));
#20998=DIRECTION('',(1.,1.22464679914735E-16,0.));
#20999=DIRECTION('center_axis',(-1.,-1.22464679914735E-16,0.));
#21000=DIRECTION('ref_axis',(1.22464679914735E-16,-1.,0.));
#21001=DIRECTION('center_axis',(-1.,-1.22464679914735E-16,0.));
#21002=DIRECTION('ref_axis',(1.22464679914735E-16,-1.,0.));
#21003=DIRECTION('center_axis',(1.,1.22464679914735E-16,0.));
#21004=DIRECTION('ref_axis',(-1.22464679914735E-16,1.,0.));
#21005=DIRECTION('',(1.,1.22464679914735E-16,0.));
#21006=DIRECTION('center_axis',(-1.,-1.22464679914735E-16,0.));
#21007=DIRECTION('ref_axis',(1.22464679914735E-16,-1.,0.));
#21008=DIRECTION('',(-1.,-1.22464679914735E-16,0.));
#21009=DIRECTION('center_axis',(-1.,-1.22464679914735E-16,0.));
#21010=DIRECTION('ref_axis',(1.22464679914735E-16,-1.,0.));
#21011=DIRECTION('center_axis',(1.,1.22464679914735E-16,0.));
#21012=DIRECTION('ref_axis',(-1.22464679914735E-16,1.,0.));
#21013=DIRECTION('',(1.,1.22464679914735E-16,0.));
#21014=DIRECTION('center_axis',(-1.,-1.22464679914735E-16,0.));
#21015=DIRECTION('ref_axis',(1.22464679914735E-16,-1.,0.));
#21016=DIRECTION('center_axis',(-1.,-1.22464679914735E-16,0.));
#21017=DIRECTION('ref_axis',(1.22464679914735E-16,-1.,0.));
#21018=DIRECTION('center_axis',(-1.,-1.22464679914735E-16,0.));
#21019=DIRECTION('ref_axis',(1.22464679914735E-16,-1.,0.));
#21020=DIRECTION('center_axis',(1.,1.22464679914735E-16,0.));
#21021=DIRECTION('ref_axis',(-1.22464679914735E-16,1.,0.));
#21022=DIRECTION('center_axis',(-1.,-1.22464679914735E-16,0.));
#21023=DIRECTION('ref_axis',(1.22464679914735E-16,-1.,0.));
#21024=DIRECTION('center_axis',(-1.,-1.22464679914735E-16,0.));
#21025=DIRECTION('ref_axis',(1.22464679914735E-16,-1.,0.));
#21026=DIRECTION('',(-1.,-1.22464679914735E-16,0.));
#21027=DIRECTION('center_axis',(1.,1.22464679914735E-16,0.));
#21028=DIRECTION('ref_axis',(-1.22464679914735E-16,1.,0.));
#21029=DIRECTION('center_axis',(-1.,-1.22464679914735E-16,0.));
#21030=DIRECTION('ref_axis',(1.22464679914735E-16,-1.,0.));
#21031=DIRECTION('center_axis',(-1.,-1.22464679914735E-16,0.));
#21032=DIRECTION('ref_axis',(1.22464679914735E-16,-1.,0.));
#21033=DIRECTION('',(-1.,-1.22464679914735E-16,0.));
#21034=DIRECTION('center_axis',(1.,1.22464679914735E-16,0.));
#21035=DIRECTION('ref_axis',(-1.22464679914735E-16,1.,0.));
#21036=DIRECTION('',(1.,1.22464679914735E-16,0.));
#21037=DIRECTION('center_axis',(1.,1.22464679914735E-16,0.));
#21038=DIRECTION('ref_axis',(-1.24344978758018E-16,1.,0.));
#21039=DIRECTION('center_axis',(-1.,-1.22464679914735E-16,0.));
#21040=DIRECTION('ref_axis',(-1.22464679914735E-16,1.,-7.99360577730113E-15));
#21041=DIRECTION('center_axis',(-8.10039603428687E-17,0.661447532458067,
-0.749991441154587));
#21042=DIRECTION('ref_axis',(-2.96250659143342E-32,-0.749991441154587,-0.661447532458067));
#21043=DIRECTION('center_axis',(3.90402550029783E-17,-0.318787874431711,
0.947826086956522));
#21044=DIRECTION('ref_axis',(-3.57000607053533E-33,-0.947826086956522,-0.318787874431711));
#21045=DIRECTION('center_axis',(1.,1.22464679914735E-16,0.));
#21046=DIRECTION('ref_axis',(-1.24344978758018E-16,1.,0.));
#21047=DIRECTION('center_axis',(-1.,-1.22464679914735E-16,0.));
#21048=DIRECTION('ref_axis',(-1.22464679914735E-16,1.,0.));
#21049=DIRECTION('center_axis',(3.90402550029783E-17,-0.318787874431711,
-0.947826086956522));
#21050=DIRECTION('ref_axis',(-3.57000607053533E-33,-0.947826086956522,0.318787874431711));
#21051=DIRECTION('center_axis',(-8.10039603428704E-17,0.661447532458081,
0.749991441154575));
#21052=DIRECTION('ref_axis',(7.37954811975299E-33,-0.749991441154575,0.661447532458081));
#21053=DIRECTION('center_axis',(1.,1.22464679914735E-16,0.));
#21054=DIRECTION('ref_axis',(-1.24344978758018E-16,1.,0.));
#21055=DIRECTION('center_axis',(1.20044215345851E-16,-0.980235406889814,
0.197834645801896));
#21056=DIRECTION('ref_axis',(-2.0076031589995E-32,-0.197834645801896,-0.980235406889814));
#21057=DIRECTION('center_axis',(-1.,-1.22464679914735E-16,0.));
#21058=DIRECTION('ref_axis',(-1.22464679914735E-16,1.,7.105427357601E-15));
#21059=DIRECTION('center_axis',(-1.20044215345851E-16,0.980235406889808,
0.197834645801926));
#21060=DIRECTION('ref_axis',(1.61897508715493E-32,0.197834645801926,-0.980235406889808));
#21061=DIRECTION('center_axis',(1.,1.22464679914735E-16,0.));
#21062=DIRECTION('ref_axis',(-1.24344978758018E-16,1.,0.));
#21063=DIRECTION('center_axis',(8.10039603428609E-17,-0.661447532458004,
-0.749991441154643));
#21064=DIRECTION('ref_axis',(7.96570883309855E-33,0.749991441154643,-0.661447532458004));
#21065=DIRECTION('center_axis',(-1.,-1.22464679914735E-16,0.));
#21066=DIRECTION('ref_axis',(-1.22464679914735E-16,1.,0.));
#21067=DIRECTION('center_axis',(-3.90402550029794E-17,0.31878787443172,
0.947826086956519));
#21068=DIRECTION('ref_axis',(2.68331918262955E-33,0.947826086956519,-0.31878787443172));
#21069=DIRECTION('center_axis',(1.,1.22464679914735E-16,0.));
#21070=DIRECTION('ref_axis',(-1.24344978758018E-16,1.,0.));
#21071=DIRECTION('center_axis',(1.,1.22464679914735E-16,0.));
#21072=DIRECTION('ref_axis',(-1.22464679914735E-16,1.,0.));
#21073=DIRECTION('center_axis',(-1.20044215345852E-16,0.980235406889816,
-0.197834645801884));
#21074=DIRECTION('ref_axis',(-2.66733220812947E-32,0.197834645801884,0.980235406889816));
#21075=DIRECTION('center_axis',(-1.,-1.22464679914735E-16,0.));
#21076=DIRECTION('ref_axis',(-1.22464679914735E-16,1.,0.));
#21077=DIRECTION('center_axis',(1.20044215345849E-16,-0.980235406889798,
-0.197834645801971));
#21078=DIRECTION('ref_axis',(-7.95464076645661E-33,-0.197834645801971,0.980235406889798));
#21079=DIRECTION('center_axis',(-1.,-1.22464679914735E-16,0.));
#21080=DIRECTION('ref_axis',(1.4210854715202E-16,-1.,0.));
#21081=DIRECTION('center_axis',(-8.10039603428687E-17,0.661447532458067,
-0.749991441154587));
#21082=DIRECTION('ref_axis',(-2.27599120852545E-32,0.749991441154587,0.661447532458068));
#21083=DIRECTION('center_axis',(1.,1.22464679914735E-16,0.));
#21084=DIRECTION('ref_axis',(1.22464679914735E-16,-1.,0.));
#21085=DIRECTION('center_axis',(3.90402550029783E-17,-0.318787874431711,
0.947826086956522));
#21086=DIRECTION('ref_axis',(1.97143231695727E-32,0.947826086956522,0.318787874431711));
#21087=DIRECTION('center_axis',(-1.,-1.22464679914735E-16,0.));
#21088=DIRECTION('ref_axis',(1.4210854715202E-16,-1.,0.));
#21089=DIRECTION('center_axis',(3.90402550029783E-17,-0.318787874431711,
-0.947826086956522));
#21090=DIRECTION('ref_axis',(1.97143231695727E-32,0.947826086956522,-0.318787874431711));
#21091=DIRECTION('center_axis',(1.,1.22464679914735E-16,0.));
#21092=DIRECTION('ref_axis',(1.22464679914735E-16,-1.,-2.66453525910038E-15));
#21093=DIRECTION('center_axis',(-8.10039603428704E-17,0.661447532458081,
0.749991441154575));
#21094=DIRECTION('ref_axis',(2.2108738618768E-32,0.749991441154575,-0.661447532458081));
#21095=DIRECTION('center_axis',(-1.,-1.22464679914735E-16,0.));
#21096=DIRECTION('ref_axis',(1.4210854715202E-16,-1.,0.));
#21097=DIRECTION('center_axis',(1.,1.22464679914735E-16,0.));
#21098=DIRECTION('ref_axis',(1.22464679914735E-16,-1.,7.105427357601E-15));
#21099=DIRECTION('center_axis',(1.20044215345851E-16,-0.980235406889814,
0.197834645801896));
#21100=DIRECTION('ref_axis',(2.0076031589995E-32,0.197834645801896,0.980235406889814));
#21101=DIRECTION('center_axis',(-1.20044215345851E-16,0.980235406889808,
0.197834645801926));
#21102=DIRECTION('ref_axis',(-1.61897508715493E-32,-0.197834645801926,0.980235406889808));
#21103=DIRECTION('center_axis',(-1.,-1.22464679914735E-16,0.));
#21104=DIRECTION('ref_axis',(1.4210854715202E-16,-1.,0.));
#21105=DIRECTION('center_axis',(1.,1.22464679914735E-16,0.));
#21106=DIRECTION('ref_axis',(1.22464679914735E-16,-1.,1.77635683940025E-15));
#21107=DIRECTION('center_axis',(8.10039603428609E-17,-0.661447532458004,
-0.749991441154643));
#21108=DIRECTION('ref_axis',(-5.20417042793042E-15,-0.749991441154643,0.661447532458004));
#21109=DIRECTION('center_axis',(-3.90402550029794E-17,0.31878787443172,
0.947826086956519));
#21110=DIRECTION('ref_axis',(-2.68331918262955E-33,-0.947826086956519,0.31878787443172));
#21111=DIRECTION('center_axis',(-1.,-1.22464679914735E-16,0.));
#21112=DIRECTION('ref_axis',(1.4210854715202E-16,-1.,0.));
#21113=DIRECTION('center_axis',(1.,1.22464679914735E-16,0.));
#21114=DIRECTION('ref_axis',(1.22464679914735E-16,-1.,0.));
#21115=DIRECTION('center_axis',(-1.20044215345852E-16,0.980235406889816,
-0.197834645801884));
#21116=DIRECTION('ref_axis',(2.66733220812947E-32,-0.197834645801884,-0.980235406889816));
#21117=DIRECTION('center_axis',(-1.,-1.22464679914735E-16,0.));
#21118=DIRECTION('ref_axis',(1.22464679914735E-16,-1.,0.));
#21119=DIRECTION('center_axis',(1.20044215345849E-16,-0.980235406889798,
-0.197834645801971));
#21120=DIRECTION('ref_axis',(7.95464076645661E-33,0.197834645801971,-0.980235406889798));
#21121=DIRECTION('center_axis',(1.,1.22464679914735E-16,0.));
#21122=DIRECTION('ref_axis',(-1.22464679914735E-16,1.,0.));
#21123=DIRECTION('center_axis',(1.,1.22464679914735E-16,0.));
#21124=DIRECTION('ref_axis',(-1.22464679914735E-16,1.,0.));
#21125=DIRECTION('center_axis',(1.,1.22464679914735E-16,0.));
#21126=DIRECTION('ref_axis',(-1.22464679914735E-16,1.,0.));
#21127=DIRECTION('center_axis',(1.,1.22464679914735E-16,0.));
#21128=DIRECTION('ref_axis',(-1.22464679914735E-16,1.,0.));
#21129=DIRECTION('center_axis',(-1.,-1.22464679914735E-16,0.));
#21130=DIRECTION('ref_axis',(-1.22464679914735E-16,1.,0.));
#21131=DIRECTION('center_axis',(-1.,-1.22464679914735E-16,0.));
#21132=DIRECTION('ref_axis',(1.22464679914735E-16,-1.,0.));
#21133=DIRECTION('',(-1.,-1.22464679914735E-16,0.));
#21134=DIRECTION('',(1.,1.22464679914735E-16,0.));
#21135=DIRECTION('center_axis',(-1.,-1.22464679914735E-16,0.));
#21136=DIRECTION('ref_axis',(1.22464679914735E-16,-1.,0.));
#21137=DIRECTION('center_axis',(-1.,-1.22464679914735E-16,0.));
#21138=DIRECTION('ref_axis',(1.22464679914735E-16,-1.,0.));
#21139=DIRECTION('center_axis',(-1.,-1.22464679914735E-16,0.));
#21140=DIRECTION('ref_axis',(1.22464679914735E-16,-1.,0.));
#21141=DIRECTION('center_axis',(1.,1.22464679914735E-16,0.));
#21142=DIRECTION('ref_axis',(1.22464679914735E-16,-1.,0.));
#21143=DIRECTION('center_axis',(-1.,-1.22464679914735E-16,0.));
#21144=DIRECTION('ref_axis',(1.22464679914735E-16,-1.,0.));
#21145=DIRECTION('center_axis',(-1.,-1.22464679914735E-16,0.));
#21146=DIRECTION('ref_axis',(1.22464679914735E-16,-1.,0.));
#21147=DIRECTION('center_axis',(-1.,-1.22464679914735E-16,0.));
#21148=DIRECTION('ref_axis',(1.22464679914735E-16,-1.,0.));
#21149=DIRECTION('center_axis',(1.,1.22464679914735E-16,0.));
#21150=DIRECTION('ref_axis',(-1.24344978758018E-16,1.,0.));
#21151=DIRECTION('center_axis',(-3.90402550029925E-17,0.318787874431827,
-0.947826086956483));
#21152=DIRECTION('ref_axis',(-6.44688282815806E-33,0.947826086956483,0.318787874431827));
#21153=DIRECTION('center_axis',(8.10039603428727E-17,-0.6614475324581,0.749991441154558));
#21154=DIRECTION('ref_axis',(-3.97296770160977E-32,0.749991441154558,0.6614475324581));
#21155=DIRECTION('center_axis',(-1.,-1.22464679914735E-16,0.));
#21156=DIRECTION('ref_axis',(1.4210854715202E-16,-1.,0.));
#21157=DIRECTION('center_axis',(-3.90402550029925E-17,0.318787874431827,
-0.947826086956483));
#21158=DIRECTION('ref_axis',(-1.26985355407412E-32,-0.947826086956483,-0.318787874431827));
#21159=DIRECTION('center_axis',(8.10039603428727E-17,-0.6614475324581,0.749991441154558));
#21160=DIRECTION('ref_axis',(3.97296770160977E-32,-0.749991441154558,-0.6614475324581));
#21161=DIRECTION('center_axis',(1.,1.22464679914735E-16,0.));
#21162=DIRECTION('ref_axis',(6.12323399573693E-17,-0.500000000000013,0.866025403784431));
#21163=DIRECTION('',(-1.,-1.22464679914735E-16,0.));
#21164=DIRECTION('center_axis',(-1.,-1.22464679914735E-16,0.));
#21165=DIRECTION('ref_axis',(-1.22464679914735E-16,1.,1.15648231731783E-15));
#21166=DIRECTION('',(1.,1.22464679914735E-16,0.));
#21167=DIRECTION('center_axis',(1.,1.22464679914735E-16,0.));
#21168=DIRECTION('ref_axis',(6.12323399573661E-17,-0.499999999999987,-0.866025403784446));
#21169=DIRECTION('',(-1.,-1.22464679914735E-16,0.));
#21170=DIRECTION('center_axis',(-1.,-1.22464679914735E-16,0.));
#21171=DIRECTION('ref_axis',(-1.22464679914735E-16,1.,1.15648231731771E-15));
#21172=DIRECTION('center_axis',(1.,1.22464679914735E-16,0.));
#21173=DIRECTION('ref_axis',(1.22464679914735E-16,-1.,-1.22464679914735E-16));
#21174=DIRECTION('',(-1.,-1.22464679914735E-16,0.));
#21175=DIRECTION('center_axis',(-1.,-1.22464679914735E-16,0.));
#21176=DIRECTION('ref_axis',(-1.22464679914735E-16,1.,8.88178419700125E-16));
#21177=DIRECTION('center_axis',(1.,0.,0.));
#21178=DIRECTION('ref_axis',(0.,-0.111847407981875,-0.99372539331937));
#21179=DIRECTION('center_axis',(0.,-0.111847407981874,-0.99372539331937));
#21180=DIRECTION('ref_axis',(0.,0.99372539331937,-0.111847407981874));
#21181=DIRECTION('center_axis',(1.,0.,0.));
#21182=DIRECTION('ref_axis',(0.,-0.111847407981875,-0.99372539331937));
#21183=DIRECTION('center_axis',(1.,1.22464679914735E-16,0.));
#21184=DIRECTION('ref_axis',(4.44089209850026E-17,-0.499999999999987,-0.866025403784446));
#21185=DIRECTION('center_axis',(0.,0.804667731009303,0.593725393319454));
#21186=DIRECTION('ref_axis',(0.,-0.593725393319454,0.804667731009303));
#21187=DIRECTION('center_axis',(1.,0.,0.));
#21188=DIRECTION('ref_axis',(0.,0.804667731009302,0.593725393319455));
#21189=DIRECTION('center_axis',(1.,0.,0.));
#21190=DIRECTION('ref_axis',(0.,0.,-1.));
#21191=DIRECTION('center_axis',(1.,0.,0.));
#21192=DIRECTION('ref_axis',(0.,0.804667731009302,0.593725393319455));
#21193=DIRECTION('center_axis',(-1.,0.,0.));
#21194=DIRECTION('ref_axis',(0.,0.,1.));
#21195=DIRECTION('center_axis',(-1.,-1.22464679914735E-16,0.));
#21196=DIRECTION('ref_axis',(1.22464679914735E-16,-1.,0.));
#21197=DIRECTION('center_axis',(1.,1.22464679914735E-16,0.));
#21198=DIRECTION('ref_axis',(-1.22464679914735E-16,1.,0.));
#21199=DIRECTION('center_axis',(-1.,0.,0.));
#21200=DIRECTION('ref_axis',(0.,0.,1.));
#21201=DIRECTION('center_axis',(1.,0.,0.));
#21202=DIRECTION('ref_axis',(0.,0.,-1.));
#21203=DIRECTION('center_axis',(1.,0.,0.));
#21204=DIRECTION('ref_axis',(0.,0.804667731009333,-0.593725393319414));
#21205=DIRECTION('center_axis',(1.,0.,0.));
#21206=DIRECTION('ref_axis',(0.,0.804667731009332,-0.593725393319415));
#21207=DIRECTION('center_axis',(-1.91085069238026E-15,0.804667731009333,
-0.593725393319414));
#21208=DIRECTION('ref_axis',(2.55801177487293E-31,0.593725393319413,0.804667731009333));
#21209=DIRECTION('center_axis',(-1.,-1.22464679914735E-16,0.));
#21210=DIRECTION('ref_axis',(0.,0.500000000000037,-0.866025403784417));
#21211=DIRECTION('center_axis',(1.62682660628867E-15,-0.11184740798194,
0.993725393319362));
#21212=DIRECTION('ref_axis',(8.0958773252926E-32,-0.993725393319362,-0.11184740798194));
#21213=DIRECTION('center_axis',(1.,0.,0.));
#21214=DIRECTION('ref_axis',(0.,-0.111847407981939,0.993725393319362));
#21215=DIRECTION('center_axis',(1.,0.,0.));
#21216=DIRECTION('ref_axis',(0.,-0.111847407981939,0.993725393319362));
#21217=DIRECTION('center_axis',(1.,1.22464679914735E-16,0.));
#21218=DIRECTION('ref_axis',(1.11949878192378E-16,-0.914140128160396,0.405398354815231));
#21219=DIRECTION('center_axis',(-1.,-1.99493199737328E-16,-8.70659703262238E-17));
#21220=DIRECTION('ref_axis',(1.99493199737328E-16,-1.,-1.51035382683644E-33));
#21221=DIRECTION('center_axis',(1.,0.,0.));
#21222=DIRECTION('ref_axis',(0.,0.,-1.));
#21223=DIRECTION('center_axis',(1.,0.,0.));
#21224=DIRECTION('ref_axis',(0.,0.916515138991152,0.400000000000037));
#21225=DIRECTION('center_axis',(1.,0.,0.));
#21226=DIRECTION('ref_axis',(0.,0.916515138991152,0.400000000000037));
#21227=DIRECTION('center_axis',(0.,0.916515138991152,0.400000000000037));
#21228=DIRECTION('ref_axis',(0.,-0.400000000000037,0.916515138991152));
#21229=DIRECTION('center_axis',(-1.,-1.22464679914735E-16,0.));
#21230=DIRECTION('ref_axis',(-1.77635683939998E-16,1.,5.67209541808933E-14));
#21231=DIRECTION('center_axis',(3.46944695195304E-16,-0.916515138991197,
0.399999999999933));
#21232=DIRECTION('ref_axis',(-7.5199079965689E-34,-0.399999999999933,-0.916515138991197));
#21233=DIRECTION('center_axis',(1.,0.,0.));
#21234=DIRECTION('ref_axis',(0.,-0.916515138991197,0.399999999999933));
#21235=DIRECTION('center_axis',(1.,0.,0.));
#21236=DIRECTION('ref_axis',(0.,-0.916515138991197,0.399999999999933));
#21237=DIRECTION('center_axis',(-1.,-1.22464679914735E-16,0.));
#21238=DIRECTION('ref_axis',(0.,0.499999999999963,0.86602540378446));
#21239=DIRECTION('center_axis',(0.,-0.111847407981704,-0.993725393319389));
#21240=DIRECTION('ref_axis',(0.,0.993725393319389,-0.111847407981704));
#21241=DIRECTION('center_axis',(2.42582538141761E-15,-0.804667731009371,
-0.593725393319361));
#21242=DIRECTION('ref_axis',(-2.98202186050019E-31,0.593725393319361,-0.804667731009371));
#21243=DIRECTION('center_axis',(1.,4.44089209850063E-16,0.));
#21244=DIRECTION('ref_axis',(0.,0.111847407981704,0.993725393319389));
#21245=DIRECTION('center_axis',(-1.,0.,0.));
#21246=DIRECTION('ref_axis',(0.,0.,1.));
#21247=DIRECTION('center_axis',(1.,0.,0.));
#21248=DIRECTION('ref_axis',(0.,-0.804667731009372,-0.593725393319361));
#21249=DIRECTION('center_axis',(-1.,0.,0.));
#21250=DIRECTION('ref_axis',(0.,0.,1.));
#21251=DIRECTION('center_axis',(1.,1.22464679914735E-16,0.));
#21252=DIRECTION('ref_axis',(9.8970484789873E-17,-0.808155338002599,-0.588969396198059));
#21253=DIRECTION('center_axis',(-1.,0.,0.));
#21254=DIRECTION('ref_axis',(0.,0.,1.));
#21255=DIRECTION('center_axis',(-1.,-1.22464679914735E-16,0.));
#21256=DIRECTION('ref_axis',(1.22464679914735E-16,-1.,0.));
#21257=DIRECTION('center_axis',(-1.,0.,0.));
#21258=DIRECTION('ref_axis',(0.,0.,1.));
#21259=DIRECTION('center_axis',(1.,0.,0.));
#21260=DIRECTION('ref_axis',(0.,0.111847407981704,0.993725393319389));
#21261=DIRECTION('center_axis',(1.,0.,0.));
#21262=DIRECTION('ref_axis',(0.,-0.804667731009372,-0.593725393319361));
#21263=DIRECTION('center_axis',(1.,0.,0.));
#21264=DIRECTION('ref_axis',(0.,-0.916515138991168,-0.400000000000001));
#21265=DIRECTION('center_axis',(1.,0.,0.));
#21266=DIRECTION('ref_axis',(0.,0.916515138991168,-0.400000000000001));
#21267=DIRECTION('center_axis',(-1.,0.,0.));
#21268=DIRECTION('ref_axis',(0.,0.,1.));
#21269=DIRECTION('center_axis',(-1.,-1.22464679914735E-16,0.));
#21270=DIRECTION('ref_axis',(-1.11949878192374E-16,0.914140128160362,0.405398354815307));
#21271=DIRECTION('center_axis',(-1.,-1.99493199737332E-16,8.70659703262165E-17));
#21272=DIRECTION('ref_axis',(1.99493199737332E-16,-1.,1.51035382683594E-33));
#21273=DIRECTION('center_axis',(1.,0.,0.));
#21274=DIRECTION('ref_axis',(0.,-0.916515138991168,-0.400000000000001));
#21275=DIRECTION('center_axis',(0.,-0.916515138991168,-0.4));
#21276=DIRECTION('ref_axis',(0.,0.4,-0.916515138991168));
#21277=DIRECTION('center_axis',(1.,0.,0.));
#21278=DIRECTION('ref_axis',(0.,0.916515138991168,-0.400000000000001));
#21279=DIRECTION('center_axis',(-1.24295563250076E-15,-0.916515138991168,
0.400000000000001));
#21280=DIRECTION('ref_axis',(7.88837516234267E-32,-0.400000000000001,-0.916515138991168));
#21281=DIRECTION('center_axis',(1.,1.22464679914735E-16,0.));
#21282=DIRECTION('ref_axis',(1.11022302462516E-16,-1.,1.22464679914735E-16));
#21283=DIRECTION('center_axis',(1.,0.,0.));
#21284=DIRECTION('ref_axis',(0.,-0.804667731009409,0.59372539331931));
#21285=DIRECTION('center_axis',(-1.,0.,0.));
#21286=DIRECTION('ref_axis',(0.,0.,1.));
#21287=DIRECTION('center_axis',(1.,4.44089209850063E-16,0.));
#21288=DIRECTION('ref_axis',(0.,0.111847407981753,-0.993725393319383));
#21289=DIRECTION('center_axis',(-1.,0.,0.));
#21290=DIRECTION('ref_axis',(0.,0.,1.));
#21291=DIRECTION('center_axis',(1.,1.22464679914735E-16,0.));
#21292=DIRECTION('ref_axis',(-1.22464679914735E-16,1.,0.));
#21293=DIRECTION('center_axis',(-1.,0.,0.));
#21294=DIRECTION('ref_axis',(0.,0.,1.));
#21295=DIRECTION('center_axis',(-1.,-1.22464679914735E-16,0.));
#21296=DIRECTION('ref_axis',(-9.89704847898782E-17,0.808155338002642,-0.588969396197999));
#21297=DIRECTION('center_axis',(-1.,-2.13362867122436E-16,-4.30616635022305E-17));
#21298=DIRECTION('ref_axis',(2.13362867122436E-16,-1.,-1.49749836094163E-34));
#21299=DIRECTION('center_axis',(1.,0.,0.));
#21300=DIRECTION('ref_axis',(0.,-0.804667731009409,0.59372539331931));
#21301=DIRECTION('center_axis',(0.,-0.804667731009409,0.59372539331931));
#21302=DIRECTION('ref_axis',(0.,-0.59372539331931,-0.804667731009409));
#21303=DIRECTION('center_axis',(1.,0.,0.));
#21304=DIRECTION('ref_axis',(0.,0.111847407981753,-0.993725393319383));
#21305=DIRECTION('center_axis',(0.,-0.111847407981753,0.993725393319383));
#21306=DIRECTION('ref_axis',(0.,-0.993725393319383,-0.111847407981753));
#21307=DIRECTION('center_axis',(1.,1.22464679914735E-16,0.));
#21308=DIRECTION('ref_axis',(4.44089209850053E-17,-0.500000000000013,0.866025403784431));
#33054=CARTESIAN_POINT('',(0.,0.,0.));
#33055=CARTESIAN_POINT('Origin',(13.,12.5000000000006,-21.6506350946113));
#33056=CARTESIAN_POINT('',(13.,16.0623523599166,-16.8226287085547));
#33057=CARTESIAN_POINT('',(13.,6.5376476400841,-22.3217195425019));
#33058=CARTESIAN_POINT('Origin',(13.,12.5000000000006,-21.6506350946113));
#33059=CARTESIAN_POINT('',(15.,17.2498031465552,-15.2132932465359));
#33060=CARTESIAN_POINT('Origin',(13.,17.2498031465552,-15.2132932465359));
#33061=CARTESIAN_POINT('',(15.,4.55019685344533,-22.5454143584654));
#33062=CARTESIAN_POINT('Origin',(15.,12.5000000000006,-21.6506350946113));
#33063=CARTESIAN_POINT('Origin',(13.,4.55019685344533,-22.5454143584654));
#33064=CARTESIAN_POINT('Origin',(-8.28173040415688E-15,21.8,7.33212111192934));
#33065=CARTESIAN_POINT('',(2.,23.695652173913,7.96969686079276));
#33066=CARTESIAN_POINT('',(2.,22.6,5.49909083394701));
#33067=CARTESIAN_POINT('Origin',(2.,21.8,7.33212111192934));
#33068=CARTESIAN_POINT('',(13.,23.695652173913,7.96969686079277));
#33069=CARTESIAN_POINT('',(-2.90188045884916E-15,23.695652173913,7.96969686079276));
#33070=CARTESIAN_POINT('',(13.,22.6,5.49909083394701));
#33071=CARTESIAN_POINT('Origin',(13.,21.8,7.33212111192934));
#33072=CARTESIAN_POINT('',(-8.37970214808867E-15,22.6,5.49909083394701));
#33073=CARTESIAN_POINT('Origin',(13.,25.,0.));
#33074=CARTESIAN_POINT('',(13.,22.6,-5.49909083394701));
#33075=CARTESIAN_POINT('Origin',(13.,25.,0.));
#33076=CARTESIAN_POINT('',(15.,21.8,7.33212111192934));
#33077=CARTESIAN_POINT('Origin',(13.,21.8,7.33212111192934));
#33078=CARTESIAN_POINT('',(15.,21.8,-7.33212111192935));
#33079=CARTESIAN_POINT('Origin',(15.,25.,0.));
#33080=CARTESIAN_POINT('Origin',(13.,21.8,-7.33212111192934));
#33081=CARTESIAN_POINT('Origin',(2.,-12.4999999999994,-21.650635094612));
#33082=CARTESIAN_POINT('',(2.,-16.0623523599161,-16.822628708555));
#33083=CARTESIAN_POINT('',(2.,-6.53764764008211,-22.3217195425024));
#33084=CARTESIAN_POINT('Origin',(2.,-12.4999999999994,-21.650635094612));
#33085=CARTESIAN_POINT('',(3.84721509691184E-15,-17.2498031465548,-15.2132932465363));
#33086=CARTESIAN_POINT('Origin',(2.,-17.2498031465548,-15.2132932465363));
#33087=CARTESIAN_POINT('',(2.29196187718278E-15,-4.55019685344333,-22.5454143584658));
#33088=CARTESIAN_POINT('Origin',(3.46944695195361E-15,-12.4999999999994,
-21.650635094612));
#33089=CARTESIAN_POINT('Origin',(2.,-4.55019685344333,-22.5454143584658));
#33090=CARTESIAN_POINT('Origin',(-2.12661045170397E-15,-21.7999999999999,
7.33212111192955));
#33091=CARTESIAN_POINT('',(13.,-22.5999999999998,5.49909083394716));
#33092=CARTESIAN_POINT('',(13.,-23.695652173913,7.969696860793));
#33093=CARTESIAN_POINT('Origin',(13.,-21.7999999999999,7.33212111192956));
#33094=CARTESIAN_POINT('',(2.00000000000001,-23.695652173913,7.969696860793));
#33095=CARTESIAN_POINT('',(2.90188045884915E-15,-23.695652173913,7.96969686079299));
#33096=CARTESIAN_POINT('',(2.,-22.5999999999998,5.49909083394716));
#33097=CARTESIAN_POINT('Origin',(2.,-21.7999999999999,7.33212111192956));
#33098=CARTESIAN_POINT('',(-2.0286387077722E-15,-22.5999999999998,5.49909083394716));
#33099=CARTESIAN_POINT('Origin',(2.00000000000001,-25.,-1.4119006205266E-12));
#33100=CARTESIAN_POINT('',(2.,-22.5999999999992,-5.49909083394971));
#33101=CARTESIAN_POINT('Origin',(2.00000000000001,-25.,-1.4119006205266E-12));
#33102=CARTESIAN_POINT('',(4.40445349811803E-15,-21.7999999999999,7.33212111192956));
#33103=CARTESIAN_POINT('Origin',(2.,-21.7999999999999,7.33212111192956));
#33104=CARTESIAN_POINT('',(4.40445349811793E-15,-21.7999999999991,-7.33212111193202));
#33105=CARTESIAN_POINT('Origin',(4.77048955893622E-15,-25.,-1.4119006205266E-12));
#33106=CARTESIAN_POINT('Origin',(2.,-21.7999999999991,-7.33212111193202));
#33107=CARTESIAN_POINT('Origin',(-4.44301704968179E-15,-4.5501968534443,
22.5454143584656));
#33108=CARTESIAN_POINT('',(13.,-6.53764764008302,22.3217195425017));
#33109=CARTESIAN_POINT('',(13.,-4.94586614504815,24.5058851722452));
#33110=CARTESIAN_POINT('Origin',(13.,-4.5501968534443,22.5454143584656));
#33111=CARTESIAN_POINT('',(2.,-4.94586614504815,24.5058851722452));
#33112=CARTESIAN_POINT('',(6.05693914354447E-16,-4.94586614504815,24.5058851722452));
#33113=CARTESIAN_POINT('',(2.,-6.53764764008303,22.3217195425017));
#33114=CARTESIAN_POINT('Origin',(2.,-4.5501968534443,22.5454143584656));
#33115=CARTESIAN_POINT('',(-4.19962452524979E-15,-6.53764764008302,22.3217195425017));
#33116=CARTESIAN_POINT('Origin',(2.,-12.5000000000006,21.6506350946099));
#33117=CARTESIAN_POINT('',(2.,-16.062352359918,16.8226287085528));
#33118=CARTESIAN_POINT('Origin',(2.,-12.5000000000006,21.6506350946099));
#33119=CARTESIAN_POINT('',(2.2919618771829E-15,-4.5501968534443,22.5454143584656));
#33120=CARTESIAN_POINT('Origin',(2.,-4.5501968534443,22.5454143584656));
#33121=CARTESIAN_POINT('',(3.84721509691208E-15,-17.2498031465568,15.2132932465341));
#33122=CARTESIAN_POINT('Origin',(3.46944695195361E-15,-12.5000000000006,
21.6506350946099));
#33123=CARTESIAN_POINT('Origin',(2.,-17.2498031465568,15.2132932465341));
#33124=CARTESIAN_POINT('Origin',(13.,12.4999999999994,21.6506350946106));
#33125=CARTESIAN_POINT('',(13.,6.53764764008235,22.321719542502));
#33126=CARTESIAN_POINT('',(13.,16.0623523599166,16.8226287085542));
#33127=CARTESIAN_POINT('Origin',(13.,12.4999999999994,21.6506350946106));
#33128=CARTESIAN_POINT('',(15.,4.55019685344361,22.5454143584657));
#33129=CARTESIAN_POINT('Origin',(13.,4.55019685344361,22.5454143584657));
#33130=CARTESIAN_POINT('',(15.,17.2498031465555,15.2132932465356));
#33131=CARTESIAN_POINT('Origin',(15.,12.4999999999994,21.6506350946106));
#33132=CARTESIAN_POINT('Origin',(13.,17.2498031465555,15.2132932465355));
#33133=CARTESIAN_POINT('Origin',(-5.96532380617912E-15,4.55019685344361,
22.5454143584657));
#33134=CARTESIAN_POINT('',(2.,4.9458661450474,24.5058851722453));
#33135=CARTESIAN_POINT('',(2.,6.53764764008234,22.321719542502));
#33136=CARTESIAN_POINT('Origin',(2.,4.55019685344361,22.5454143584657));
#33137=CARTESIAN_POINT('',(13.,4.9458661450474,24.5058851722453));
#33138=CARTESIAN_POINT('',(-6.05693914354355E-16,4.9458661450474,24.5058851722453));
#33139=CARTESIAN_POINT('Origin',(13.,4.55019685344361,22.5454143584657));
#33140=CARTESIAN_POINT('',(-6.20871633061112E-15,6.53764764008235,22.321719542502));
#33141=CARTESIAN_POINT('Origin',(-3.46944695195361E-15,-12.5000000000006,
21.6506350946099));
#33142=CARTESIAN_POINT('',(13.,-16.062352359918,16.8226287085528));
#33143=CARTESIAN_POINT('',(-3.03318461045284E-15,-16.062352359918,16.8226287085528));
#33144=CARTESIAN_POINT('Origin',(13.,-12.5000000000006,21.6506350946099));
#33145=CARTESIAN_POINT('Origin',(-1.73472347597681E-15,-25.,-1.4119006205266E-12));
#33146=CARTESIAN_POINT('',(13.,-22.5999999999992,-5.49909083394971));
#33147=CARTESIAN_POINT('',(-2.02863870777227E-15,-22.5999999999992,-5.49909083394972));
#33148=CARTESIAN_POINT('Origin',(13.,-25.,-1.4119006205266E-12));
#33149=CARTESIAN_POINT('Origin',(-3.46944695195361E-15,-12.4999999999994,
-21.650635094612));
#33150=CARTESIAN_POINT('',(13.,-6.53764764008211,-22.3217195425024));
#33151=CARTESIAN_POINT('',(-4.19962452524975E-15,-6.53764764008211,-22.3217195425024));
#33152=CARTESIAN_POINT('',(13.,-16.0623523599161,-16.822628708555));
#33153=CARTESIAN_POINT('Origin',(13.,-12.4999999999994,-21.650635094612));
#33154=CARTESIAN_POINT('',(-3.03318461045291E-15,-16.0623523599161,-16.822628708555));
#33155=CARTESIAN_POINT('Origin',(0.,0.,0.));
#33156=CARTESIAN_POINT('',(30.,5.,-6.12323399573676E-16));
#33157=CARTESIAN_POINT('Origin',(30.,3.67394039744206E-15,0.));
#33158=CARTESIAN_POINT('',(18.,5.,-6.12323399573676E-16));
#33159=CARTESIAN_POINT('',(-6.12323399573676E-16,5.,-6.12323399573676E-16));
#33160=CARTESIAN_POINT('Origin',(18.,2.20436423846524E-15,0.));
#33161=CARTESIAN_POINT('Origin',(0.,0.,0.));
#33162=CARTESIAN_POINT('',(15.,12.5,-1.53080849893419E-15));
#33163=CARTESIAN_POINT('Origin',(15.,1.83697019872103E-15,0.));
#33164=CARTESIAN_POINT('',(30.,12.5,-1.53080849893419E-15));
#33165=CARTESIAN_POINT('',(-1.53080849893419E-15,12.5,-1.53080849893419E-15));
#33166=CARTESIAN_POINT('Origin',(30.,3.67394039744206E-15,0.));
#33167=CARTESIAN_POINT('Origin',(0.,0.,0.));
#33168=CARTESIAN_POINT('',(2.,18.7497860288644,-16.536188311452));
#33169=CARTESIAN_POINT('',(2.,23.695652173913,-7.96969686079276));
#33170=CARTESIAN_POINT('Origin',(2.,2.44929359829471E-16,0.));
#33171=CARTESIAN_POINT('',(13.,23.695652173913,-7.96969686079276));
#33172=CARTESIAN_POINT('',(-2.90188045884916E-15,23.695652173913,-7.96969686079276));
#33173=CARTESIAN_POINT('',(13.,18.7497860288644,-16.536188311452));
#33174=CARTESIAN_POINT('Origin',(13.,1.59204083889156E-15,0.));
#33175=CARTESIAN_POINT('',(-2.29618654449465E-15,18.7497860288644,-16.536188311452));
#33176=CARTESIAN_POINT('Origin',(0.,0.,0.));
#33177=CARTESIAN_POINT('',(2.,18.7497860288647,16.5361883114517));
#33178=CARTESIAN_POINT('Origin',(2.,2.44929359829471E-16,0.));
#33179=CARTESIAN_POINT('',(13.,18.7497860288647,16.5361883114517));
#33180=CARTESIAN_POINT('',(-2.29618654449469E-15,18.7497860288647,16.5361883114517));
#33181=CARTESIAN_POINT('Origin',(13.,1.59204083889156E-15,0.));
#33182=CARTESIAN_POINT('Origin',(0.,0.,0.));
#33183=CARTESIAN_POINT('Origin',(13.,1.59204083889156E-15,0.));
#33184=CARTESIAN_POINT('Origin',(2.,2.44929359829471E-16,0.));
#33185=CARTESIAN_POINT('Origin',(0.,0.,0.));
#33186=CARTESIAN_POINT('',(13.,-18.7497860288661,16.5361883114501));
#33187=CARTESIAN_POINT('Origin',(13.,1.59204083889156E-15,0.));
#33188=CARTESIAN_POINT('',(2.,-18.7497860288661,16.5361883114501));
#33189=CARTESIAN_POINT('',(2.29618654449486E-15,-18.7497860288661,16.5361883114501));
#33190=CARTESIAN_POINT('Origin',(2.,2.44929359829471E-16,0.));
#33191=CARTESIAN_POINT('Origin',(0.,0.,0.));
#33192=CARTESIAN_POINT('',(13.,-18.749786028864,-16.5361883114525));
#33193=CARTESIAN_POINT('',(13.,-23.6956521739121,-7.96969686079567));
#33194=CARTESIAN_POINT('Origin',(13.,1.59204083889156E-15,0.));
#33195=CARTESIAN_POINT('',(2.00000000000001,-23.6956521739121,-7.96969686079567));
#33196=CARTESIAN_POINT('',(2.90188045884904E-15,-23.6956521739121,-7.96969686079567));
#33197=CARTESIAN_POINT('',(2.,-18.7497860288639,-16.5361883114525));
#33198=CARTESIAN_POINT('Origin',(2.,2.44929359829471E-16,0.));
#33199=CARTESIAN_POINT('',(2.2961865444946E-15,-18.7497860288639,-16.5361883114525));
#33200=CARTESIAN_POINT('Origin',(2.,2.44929359829471E-16,0.));
#33201=CARTESIAN_POINT('',(-3.77768144958305E-16,17.2498031465555,15.2132932465355));
#33202=CARTESIAN_POINT('',(-9.35006546164422E-16,21.8,7.33212111192934));
#33203=CARTESIAN_POINT('Origin',(1.73472347597681E-15,2.40741243048404E-31,
0.));
#33204=CARTESIAN_POINT('Origin',(2.,17.2498031465555,15.2132932465355));
#33205=CARTESIAN_POINT('Origin',(2.,21.8,7.33212111192934));
#33206=CARTESIAN_POINT('Origin',(2.,2.44929359829471E-16,0.));
#33207=CARTESIAN_POINT('',(-9.35006546164422E-16,21.8,-7.33212111192934));
#33208=CARTESIAN_POINT('',(-3.77768144958272E-16,17.2498031465552,-15.2132932465359));
#33209=CARTESIAN_POINT('Origin',(1.73472347597681E-15,2.40741243048404E-31,
0.));
#33210=CARTESIAN_POINT('Origin',(2.,21.8,-7.33212111192934));
#33211=CARTESIAN_POINT('Origin',(2.,17.2498031465552,-15.2132932465359));
#33212=CARTESIAN_POINT('Origin',(2.,2.44929359829471E-16,0.));
#33213=CARTESIAN_POINT('',(1.1774850747708E-15,4.55019685344361,22.5454143584657));
#33214=CARTESIAN_POINT('Origin',(2.,4.55019685344361,22.5454143584657));
#33215=CARTESIAN_POINT('Origin',(1.73472347597681E-15,2.40741243048404E-31,
0.));
#33216=CARTESIAN_POINT('Origin',(2.,-4.5501968534443,22.5454143584656));
#33217=CARTESIAN_POINT('Origin',(2.,2.44929359829471E-16,0.));
#33218=CARTESIAN_POINT('Origin',(2.,-17.2498031465568,15.2132932465341));
#33219=CARTESIAN_POINT('Origin',(1.73472347597681E-15,2.40741243048404E-31,
0.));
#33220=CARTESIAN_POINT('Origin',(2.,-21.7999999999999,7.33212111192956));
#33221=CARTESIAN_POINT('Origin',(2.,2.44929359829471E-16,0.));
#33222=CARTESIAN_POINT('',(2.,-4.9458661450471,-24.5058851722454));
#33223=CARTESIAN_POINT('',(2.,4.94586614504927,-24.505885172245));
#33224=CARTESIAN_POINT('Origin',(2.,2.44929359829471E-16,0.));
#33225=CARTESIAN_POINT('Origin',(2.,-4.55019685344333,-22.5454143584658));
#33226=CARTESIAN_POINT('',(1.17748507477059E-15,4.55019685344533,-22.5454143584654));
#33227=CARTESIAN_POINT('Origin',(1.73472347597681E-15,2.40741243048404E-31,
0.));
#33228=CARTESIAN_POINT('Origin',(2.,4.55019685344533,-22.5454143584654));
#33229=CARTESIAN_POINT('Origin',(13.,1.59204083889156E-15,0.));
#33230=CARTESIAN_POINT('Origin',(13.,17.2498031465555,15.2132932465355));
#33231=CARTESIAN_POINT('Origin',(15.,1.83697019872103E-15,0.));
#33232=CARTESIAN_POINT('Origin',(13.,21.8,7.33212111192934));
#33233=CARTESIAN_POINT('Origin',(13.,1.59204083889156E-15,0.));
#33234=CARTESIAN_POINT('Origin',(13.,21.8,-7.33212111192934));
#33235=CARTESIAN_POINT('Origin',(15.,1.83697019872103E-15,0.));
#33236=CARTESIAN_POINT('Origin',(13.,17.2498031465552,-15.2132932465359));
#33237=CARTESIAN_POINT('Origin',(13.,1.59204083889156E-15,0.));
#33238=CARTESIAN_POINT('',(15.,-4.5501968534443,22.5454143584656));
#33239=CARTESIAN_POINT('Origin',(15.,1.83697019872103E-15,0.));
#33240=CARTESIAN_POINT('Origin',(13.,4.55019685344361,22.5454143584657));
#33241=CARTESIAN_POINT('Origin',(13.,-4.5501968534443,22.5454143584656));
#33242=CARTESIAN_POINT('Origin',(13.,1.59204083889156E-15,0.));
#33243=CARTESIAN_POINT('',(15.,-17.2498031465568,15.2132932465341));
#33244=CARTESIAN_POINT('',(15.,-21.7999999999999,7.33212111192955));
#33245=CARTESIAN_POINT('Origin',(15.,1.83697019872103E-15,0.));
#33246=CARTESIAN_POINT('Origin',(13.,-17.2498031465568,15.2132932465341));
#33247=CARTESIAN_POINT('Origin',(13.,-21.7999999999999,7.33212111192956));
#33248=CARTESIAN_POINT('Origin',(13.,1.59204083889156E-15,0.));
#33249=CARTESIAN_POINT('',(15.,-4.55019685344333,-22.5454143584658));
#33250=CARTESIAN_POINT('Origin',(15.,1.83697019872103E-15,0.));
#33251=CARTESIAN_POINT('',(13.,-4.94586614504711,-24.5058851722454));
#33252=CARTESIAN_POINT('Origin',(13.,-4.55019685344333,-22.5454143584658));
#33253=CARTESIAN_POINT('',(13.,4.94586614504927,-24.505885172245));
#33254=CARTESIAN_POINT('Origin',(13.,1.59204083889156E-15,0.));
#33255=CARTESIAN_POINT('Origin',(13.,4.55019685344533,-22.5454143584654));
#33256=CARTESIAN_POINT('Origin',(1.53080849893419E-15,1.87469972832732E-31,
0.));
#33257=CARTESIAN_POINT('Origin',(0.,12.4999999999994,21.6506350946106));
#33258=CARTESIAN_POINT('Origin',(-1.30104260698261E-15,25.,0.));
#33259=CARTESIAN_POINT('Origin',(0.,12.5000000000006,-21.6506350946113));
#33260=CARTESIAN_POINT('Origin',(1.73472347597681E-15,2.40741243048404E-31,
0.));
#33261=CARTESIAN_POINT('Origin',(0.,0.,0.));
#33262=CARTESIAN_POINT('',(6.05693914354321E-16,-4.94586614504712,-24.5058851722454));
#33263=CARTESIAN_POINT('',(-6.05693914354585E-16,4.94586614504927,-24.505885172245));
#33264=CARTESIAN_POINT('Origin',(15.,25.,0.));
#33265=CARTESIAN_POINT('Origin',(15.,-12.5000000000006,21.6506350946099));
#33266=CARTESIAN_POINT('',(15.,-21.7999999999991,-7.33212111193202));
#33267=CARTESIAN_POINT('Origin',(15.,-25.,-1.4119006205266E-12));
#33268=CARTESIAN_POINT('',(15.,-17.2498031465548,-15.2132932465363));
#33269=CARTESIAN_POINT('Origin',(15.,1.83697019872103E-15,0.));
#33270=CARTESIAN_POINT('Origin',(15.,-12.4999999999994,-21.650635094612));
#33271=CARTESIAN_POINT('Origin',(30.,12.5,0.));
#33272=CARTESIAN_POINT('Origin',(18.,5.,0.));
#33273=CARTESIAN_POINT('Origin',(2.,2.44929359829471E-16,0.));
#33274=CARTESIAN_POINT('Origin',(2.,-21.7999999999991,-7.33212111193202));
#33275=CARTESIAN_POINT('Origin',(2.,-17.2498031465548,-15.2132932465363));
#33276=CARTESIAN_POINT('Origin',(13.,1.59204083889156E-15,0.));
#33277=CARTESIAN_POINT('Origin',(13.,-21.7999999999991,-7.33212111193202));
#33278=CARTESIAN_POINT('Origin',(13.,-17.2498031465548,-15.2132932465363));
#33279=CARTESIAN_POINT('Origin',(-6.93889390390723E-15,12.5000000000006,
-21.6506350946113));
#33280=CARTESIAN_POINT('',(2.,6.5376476400841,-22.3217195425019));
#33281=CARTESIAN_POINT('',(-6.20871633061119E-15,6.5376476400841,-22.3217195425019));
#33282=CARTESIAN_POINT('',(2.,16.0623523599166,-16.8226287085547));
#33283=CARTESIAN_POINT('Origin',(2.,12.5000000000006,-21.6506350946113));
#33284=CARTESIAN_POINT('',(-7.37515624540784E-15,16.0623523599166,-16.8226287085547));
#33285=CARTESIAN_POINT('Origin',(-6.93889390390723E-15,12.4999999999994,
21.6506350946106));
#33286=CARTESIAN_POINT('',(2.,16.0623523599166,16.8226287085542));
#33287=CARTESIAN_POINT('',(-7.37515624540799E-15,16.0623523599166,16.8226287085542));
#33288=CARTESIAN_POINT('Origin',(2.,12.4999999999994,21.6506350946106));
#33289=CARTESIAN_POINT('Origin',(-8.67361737988404E-15,25.,0.));
#33290=CARTESIAN_POINT('',(2.,22.6,-5.49909083394701));
#33291=CARTESIAN_POINT('',(-8.37970214808867E-15,22.6,-5.49909083394701));
#33292=CARTESIAN_POINT('Origin',(2.,25.,0.));
#33293=CARTESIAN_POINT('Origin',(2.,4.55019685344361,22.5454143584657));
#33294=CARTESIAN_POINT('Origin',(2.,4.55019685344361,22.5454143584657));
#33295=CARTESIAN_POINT('Origin',(13.,4.55019685344361,22.5454143584657));
#33296=CARTESIAN_POINT('Origin',(2.,12.4999999999994,21.6506350946106));
#33297=CARTESIAN_POINT('Origin',(2.,17.2498031465555,15.2132932465355));
#33298=CARTESIAN_POINT('Origin',(2.,17.2498031465555,15.2132932465355));
#33299=CARTESIAN_POINT('Origin',(2.,17.2498031465555,15.2132932465355));
#33300=CARTESIAN_POINT('Origin',(13.,17.2498031465555,15.2132932465355));
#33301=CARTESIAN_POINT('Origin',(13.,17.2498031465555,15.2132932465355));
#33302=CARTESIAN_POINT('Origin',(-7.52057702590823E-15,17.2498031465555,
15.2132932465355));
#33303=CARTESIAN_POINT('Origin',(-2.88776382995261E-15,-17.2498031465568,
15.2132932465341));
#33304=CARTESIAN_POINT('Origin',(2.,-17.2498031465568,15.2132932465341));
#33305=CARTESIAN_POINT('Origin',(13.,-17.2498031465568,15.2132932465341));
#33306=CARTESIAN_POINT('Origin',(2.,-17.2498031465568,15.2132932465341));
#33307=CARTESIAN_POINT('Origin',(13.,-17.2498031465568,15.2132932465341));
#33308=CARTESIAN_POINT('Origin',(13.,-17.2498031465568,15.2132932465341));
#33309=CARTESIAN_POINT('Origin',(13.,-12.5000000000006,21.6506350946099));
#33310=CARTESIAN_POINT('Origin',(13.,-4.5501968534443,22.5454143584656));
#33311=CARTESIAN_POINT('Origin',(2.,-4.5501968534443,22.5454143584656));
#33312=CARTESIAN_POINT('Origin',(13.,-4.5501968534443,22.5454143584656));
#33313=CARTESIAN_POINT('Origin',(-2.12661045170407E-15,-21.7999999999991,
-7.33212111193201));
#33314=CARTESIAN_POINT('Origin',(2.,-21.7999999999991,-7.33212111193201));
#33315=CARTESIAN_POINT('Origin',(13.,-21.7999999999991,-7.33212111193202));
#33316=CARTESIAN_POINT('Origin',(2.,-21.7999999999991,-7.33212111193202));
#33317=CARTESIAN_POINT('Origin',(13.,-21.7999999999991,-7.33212111193202));
#33318=CARTESIAN_POINT('Origin',(13.,-21.7999999999991,-7.33212111193202));
#33319=CARTESIAN_POINT('Origin',(13.,-25.,-1.4119006205266E-12));
#33320=CARTESIAN_POINT('Origin',(13.,-21.7999999999999,7.33212111192956));
#33321=CARTESIAN_POINT('Origin',(2.,-21.7999999999999,7.33212111192956));
#33322=CARTESIAN_POINT('Origin',(13.,-21.7999999999999,7.33212111192956));
#33323=CARTESIAN_POINT('Origin',(13.,-12.4999999999994,-21.650635094612));
#33324=CARTESIAN_POINT('Origin',(13.,-4.55019685344333,-22.5454143584658));
#33325=CARTESIAN_POINT('Origin',(13.,-17.2498031465548,-15.2132932465363));
#33326=CARTESIAN_POINT('Origin',(13.,-4.55019685344333,-22.5454143584658));
#33327=CARTESIAN_POINT('Origin',(13.,-4.55019685344333,-22.5454143584658));
#33328=CARTESIAN_POINT('Origin',(13.,-17.2498031465548,-15.2132932465363));
#33329=CARTESIAN_POINT('Origin',(13.,-17.2498031465548,-15.2132932465363));
#33330=CARTESIAN_POINT('Origin',(-4.44301704968176E-15,-4.55019685344334,
-22.5454143584658));
#33331=CARTESIAN_POINT('Origin',(2.,-4.55019685344334,-22.5454143584658));
#33332=CARTESIAN_POINT('Origin',(-2.8877638299527E-15,-17.2498031465548,
-15.2132932465363));
#33333=CARTESIAN_POINT('Origin',(2.,-17.2498031465548,-15.2132932465363));
#33334=CARTESIAN_POINT('Origin',(2.,-4.55019685344333,-22.5454143584658));
#33335=CARTESIAN_POINT('Origin',(2.,-17.2498031465548,-15.2132932465363));
#33336=CARTESIAN_POINT('Origin',(13.,21.8,7.33212111192934));
#33337=CARTESIAN_POINT('Origin',(13.,21.8,-7.33212111192934));
#33338=CARTESIAN_POINT('Origin',(13.,21.8,-7.33212111192934));
#33339=CARTESIAN_POINT('Origin',(-8.28173040415688E-15,21.8,-7.33212111192934));
#33340=CARTESIAN_POINT('Origin',(2.,21.8,-7.33212111192934));
#33341=CARTESIAN_POINT('Origin',(2.,21.8,7.33212111192934));
#33342=CARTESIAN_POINT('Origin',(2.,21.8,7.33212111192934));
#33343=CARTESIAN_POINT('Origin',(2.,21.8,-7.33212111192934));
#33344=CARTESIAN_POINT('Origin',(2.,21.8,-7.33212111192934));
#33345=CARTESIAN_POINT('Origin',(2.,25.,0.));
#33346=CARTESIAN_POINT('Origin',(13.,17.2498031465552,-15.2132932465359));
#33347=CARTESIAN_POINT('Origin',(13.,17.2498031465552,-15.2132932465359));
#33348=CARTESIAN_POINT('Origin',(13.,4.55019685344533,-22.5454143584654));
#33349=CARTESIAN_POINT('Origin',(13.,4.55019685344533,-22.5454143584654));
#33350=CARTESIAN_POINT('Origin',(-7.52057702590804E-15,17.2498031465552,
-15.2132932465359));
#33351=CARTESIAN_POINT('Origin',(2.,17.2498031465552,-15.2132932465359));
#33352=CARTESIAN_POINT('Origin',(-5.96532380617918E-15,4.55019685344533,
-22.5454143584654));
#33353=CARTESIAN_POINT('Origin',(2.,4.55019685344533,-22.5454143584654));
#33354=CARTESIAN_POINT('Origin',(2.,17.2498031465552,-15.2132932465359));
#33355=CARTESIAN_POINT('Origin',(2.,17.2498031465552,-15.2132932465359));
#33356=CARTESIAN_POINT('Origin',(2.,4.55019685344533,-22.5454143584654));
#33357=CARTESIAN_POINT('Origin',(2.,4.55019685344533,-22.5454143584654));
#33358=CARTESIAN_POINT('Origin',(2.,12.5000000000006,-21.6506350946113));
#38617=UNCERTAINTY_MEASURE_WITH_UNIT(LENGTH_MEASURE(0.01),#38636,
'DISTANCE_ACCURACY_VALUE',
'Maximum model space distance between geometric entities at asserted c
onnectivities');
#38619=UNCERTAINTY_MEASURE_WITH_UNIT(LENGTH_MEASURE(0.01),#38636,
'DISTANCE_ACCURACY_VALUE',
'Maximum model space distance between geometric entities at asserted c
onnectivities');
#38633=(
GEOMETRIC_REPRESENTATION_CONTEXT(3)
GLOBAL_UNCERTAINTY_ASSIGNED_CONTEXT((#38617))
GLOBAL_UNIT_ASSIGNED_CONTEXT((#38636,#38638,#38639))
REPRESENTATION_CONTEXT('','3D')
);
#38635=(
GEOMETRIC_REPRESENTATION_CONTEXT(3)
GLOBAL_UNCERTAINTY_ASSIGNED_CONTEXT((#38619))
GLOBAL_UNIT_ASSIGNED_CONTEXT((#38636,#38638,#38639))
REPRESENTATION_CONTEXT('','3D')
);
#38636=(
LENGTH_UNIT()
NAMED_UNIT(*)
SI_UNIT(.MILLI.,.METRE.)
);
#38638=(
NAMED_UNIT(*)
PLANE_ANGLE_UNIT()
SI_UNIT($,.RADIAN.)
);
#38639=(
NAMED_UNIT(*)
SI_UNIT($,.STERADIAN.)
SOLID_ANGLE_UNIT()
);
#38653=SHAPE_DEFINITION_REPRESENTATION(#38668,#38697);
#38668=PRODUCT_DEFINITION_SHAPE('',$,#38713);
#38697=SHAPE_REPRESENTATION('',(#18244),#38633);
#38699=PRODUCT_DEFINITION_CONTEXT('part definition',#38746,'design');
#38713=PRODUCT_DEFINITION('Star Knob','Star Knob',#38728,#38699);
#38728=PRODUCT_DEFINITION_FORMATION('',$,#38761);
#38746=APPLICATION_CONTEXT(
'Core Data for Automotive Mechanical Design Process');
#38747=PRODUCT_CONTEXT('part definition',#38746,'mechanical');
#38761=PRODUCT('Star Knob','Star Knob',$,(#38747));
#38765=PRESENTATION_STYLE_ASSIGNMENT((#38772));
#38772=SURFACE_STYLE_USAGE(.BOTH.,#38779);
#38779=SURFACE_SIDE_STYLE('',(#38786));
#38786=SURFACE_STYLE_FILL_AREA(#38793);
#38793=FILL_AREA_STYLE('Opaque(227,224,212)',(#38800));
#38800=FILL_AREA_STYLE_COLOUR('Opaque(227,224,212)',#38807);
#38807=COLOUR_RGB('Opaque(227,224,212)',0.890196078431372,0.87843137254902,
0.831372549019608);
ENDSEC;
END-ISO-10303-21;
